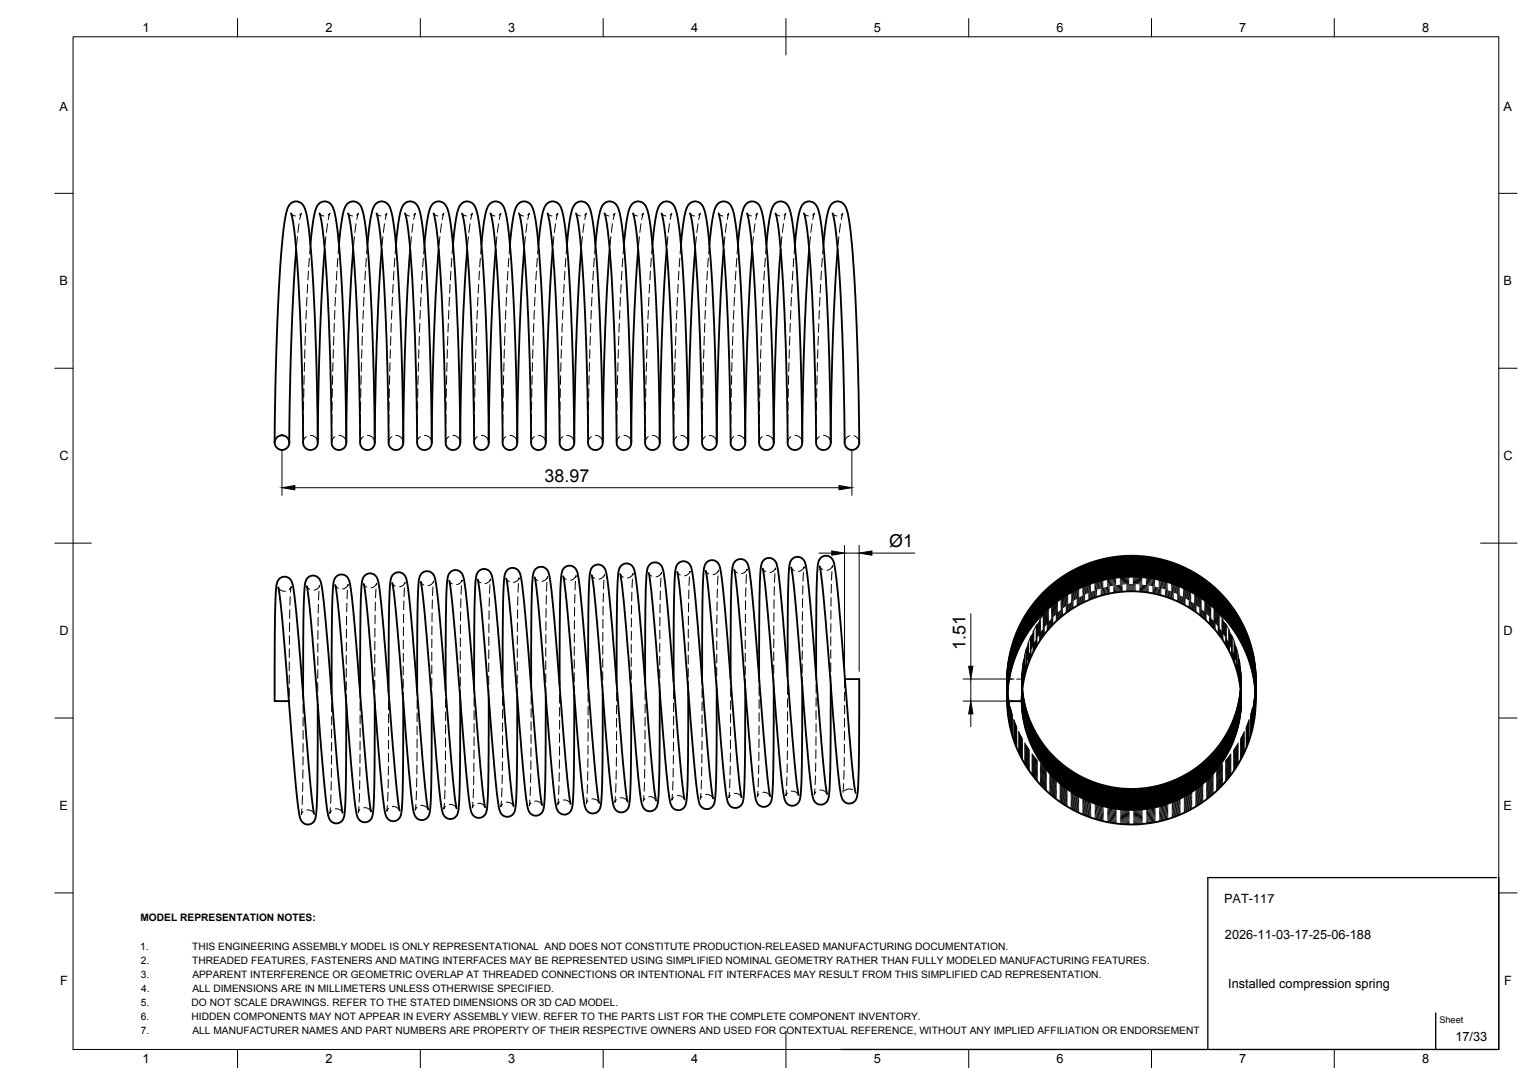
ISO-10303-21;
HEADER;
/* Generated by software containing ST-Developer
 * from STEP Tools, Inc. (www.steptools.com) 
 */

FILE_DESCRIPTION(
/* description */ ('Counterbalanced vertical column'),
/* implementation_level */ '2;1');

FILE_NAME(
/* name */ 'Installed compression spring.step',
/* time_stamp */ '2026-10-29T16:47:22-07:00',
/* author */ (''),
/* organization */ (''),
/* preprocessor_version */ 'ST-DEVELOPER v20.2',
/* originating_system */ 'Autodesk Translation Framework v15.17.0.0',
/* authorisation */ '');

FILE_SCHEMA (('AUTOMOTIVE_DESIGN { 1 0 10303 214 3 1 1 }'));
ENDSEC;

DATA;
#10=MECHANICAL_DESIGN_GEOMETRIC_PRESENTATION_REPRESENTATION('',(#364),#15040);
#278=B_SPLINE_CURVE_WITH_KNOTS('',3,(#13224,#13225,#13226,#13227,#13228,
#13229,#13230,#13231,#13232,#13233,#13234,#13235,#13236,#13237,#13238,#13239,
#13240,#13241,#13242,#13243,#13244,#13245,#13246,#13247,#13248,#13249,#13250,
#13251,#13252,#13253,#13254,#13255,#13256,#13257,#13258,#13259,#13260,#13261,
#13262,#13263,#13264,#13265,#13266,#13267,#13268,#13269,#13270,#13271,#13272,
#13273,#13274,#13275,#13276,#13277,#13278,#13279,#13280,#13281,#13282,#13283,
#13284,#13285,#13286,#13287,#13288,#13289,#13290,#13291,#13292,#13293,#13294,
#13295,#13296,#13297,#13298,#13299,#13300,#13301,#13302,#13303,#13304,#13305,
#13306,#13307,#13308,#13309,#13310,#13311,#13312,#13313,#13314,#13315,#13316,
#13317,#13318,#13319,#13320,#13321,#13322,#13323,#13324,#13325,#13326,#13327,
#13328,#13329,#13330,#13331,#13332,#13333,#13334,#13335,#13336,#13337,#13338,
#13339,#13340,#13341,#13342,#13343,#13344,#13345,#13346,#13347,#13348,#13349,
#13350,#13351,#13352,#13353,#13354,#13355,#13356,#13357,#13358,#13359,#13360,
#13361,#13362,#13363,#13364,#13365,#13366,#13367,#13368,#13369,#13370,#13371,
#13372,#13373,#13374,#13375,#13376,#13377,#13378,#13379,#13380,#13381,#13382,
#13383,#13384,#13385,#13386,#13387,#13388,#13389,#13390,#13391,#13392,#13393,
#13394,#13395,#13396,#13397,#13398,#13399,#13400,#13401,#13402,#13403,#13404,
#13405,#13406,#13407,#13408,#13409,#13410,#13411,#13412,#13413,#13414,#13415,
#13416,#13417,#13418,#13419,#13420,#13421,#13422,#13423,#13424,#13425,#13426,
#13427,#13428,#13429,#13430,#13431,#13432,#13433,#13434,#13435,#13436,#13437,
#13438,#13439,#13440,#13441,#13442,#13443,#13444,#13445,#13446,#13447,#13448,
#13449,#13450,#13451,#13452,#13453,#13454,#13455,#13456,#13457,#13458,#13459,
#13460,#13461,#13462,#13463),.UNSPECIFIED.,.F.,.F.,(4,1,1,1,1,1,1,1,1,1,
1,1,1,1,1,1,1,1,1,1,1,1,1,1,1,1,1,1,1,1,1,1,1,1,1,1,1,1,1,1,1,1,1,1,1,1,
1,1,1,1,1,1,1,1,1,1,1,1,1,1,1,1,1,1,1,1,1,1,1,1,1,1,1,1,1,1,1,1,1,1,1,1,
1,1,1,1,1,1,1,1,1,1,1,1,1,1,1,1,1,1,1,1,1,1,1,1,1,1,1,1,1,1,1,1,1,1,1,1,
1,1,1,1,1,1,1,1,1,1,1,1,1,1,1,1,1,1,1,1,1,1,1,1,1,1,1,1,1,1,1,1,1,1,1,1,
1,1,1,1,1,1,1,1,1,1,1,1,1,1,1,1,1,1,1,1,1,1,1,1,1,1,1,1,1,1,1,1,1,1,1,1,
1,1,1,1,1,1,1,1,1,1,1,1,1,1,1,1,1,1,1,1,1,1,1,1,1,1,1,1,1,1,1,1,1,1,1,1,
1,1,1,1,1,1,1,1,1,1,1,4),(0.,0.00446428571428571,0.00892857142857143,0.0133928571428571,
0.0178571428571429,0.0223214285714286,0.0267857142857143,0.03125,0.0357142857142857,
0.0401785714285714,0.0446428571428571,0.0491071428571428,0.0513392857142857,
0.0535714285714286,0.0580357142857143,0.0625,0.0669642857142857,0.0714285714285714,
0.0758928571428571,0.0803571428571428,0.0848214285714286,0.0892857142857143,
0.09375,0.0982142857142857,0.102678571428571,0.107142857142857,0.111607142857143,
0.116071428571429,0.120535714285714,0.125,0.129464285714286,0.133928571428571,
0.136160714285714,0.138392857142857,0.142857142857143,0.146825396825397,
0.150793650793651,0.154761904761905,0.158730158730159,0.162698412698413,
0.166666666666667,0.170634920634921,0.174603174603175,0.17989417989418,
0.185185185185185,0.19047619047619,0.194444444444444,0.198412698412698,
0.202380952380952,0.206349206349206,0.21031746031746,0.214285714285714,
0.218253968253968,0.220238095238095,0.222222222222222,0.226190476190476,
0.23015873015873,0.234126984126984,0.238095238095238,0.241071428571429,
0.244047619047619,0.247023809523809,0.25,0.25297619047619,0.255952380952381,
0.258928571428571,0.261904761904762,0.267857142857143,0.273809523809524,
0.279761904761905,0.285714285714286,0.291666666666667,0.297619047619048,
0.303571428571429,0.30952380952381,0.31547619047619,0.321428571428571,0.327380952380952,
0.333333333333333,0.339285714285714,0.345238095238095,0.351190476190476,
0.357142857142857,0.363095238095238,0.369047619047619,0.375,0.380952380952381,
0.386904761904762,0.392857142857143,0.398809523809524,0.404761904761905,
0.407738095238095,0.410714285714286,0.413690476190476,0.416666666666667,
0.419642857142857,0.422619047619048,0.425595238095238,0.428571428571429,
0.433035714285714,0.4375,0.441964285714286,0.446428571428571,0.450892857142857,
0.455357142857143,0.459821428571429,0.464285714285714,0.46875,0.473214285714286,
0.477678571428571,0.482142857142857,0.486607142857143,0.491071428571429,
0.495535714285714,0.5,0.504464285714286,0.508928571428571,0.513392857142857,
0.517857142857143,0.522321428571428,0.526785714285714,0.53125,0.535714285714286,
0.540178571428571,0.544642857142857,0.549107142857143,0.553571428571429,
0.558035714285714,0.5625,0.566964285714286,0.571428571428571,0.575892857142857,
0.580357142857143,0.584821428571428,0.589285714285714,0.59375,0.598214285714286,
0.602678571428571,0.607142857142857,0.611607142857143,0.616071428571429,
0.620535714285714,0.625,0.627232142857143,0.629464285714286,0.633928571428571,
0.638392857142857,0.642857142857143,0.645833333333333,0.648809523809524,
0.651785714285714,0.654761904761905,0.657738095238095,0.660714285714286,
0.663690476190476,0.666666666666667,0.66765873015873,0.670634920634921,
0.674603174603175,0.678571428571428,0.683035714285714,0.6875,0.691964285714286,
0.696428571428571,0.700892857142857,0.705357142857143,0.709821428571428,
0.714285714285714,0.717261904761905,0.720238095238095,0.723214285714286,
0.726190476190476,0.729166666666667,0.732142857142857,0.735119047619047,
0.738095238095238,0.744047619047619,0.75,0.755952380952381,0.761904761904762,
0.767857142857143,0.773809523809524,0.779761904761905,0.785714285714286,
0.78968253968254,0.793650793650793,0.797619047619047,0.801587301587302,
0.805555555555555,0.809523809523809,0.8125,0.81547619047619,0.818452380952381,
0.821428571428571,0.824404761904762,0.827380952380952,0.833333333333333,
0.836309523809524,0.839285714285714,0.842261904761905,0.845238095238095,
0.848214285714286,0.851190476190476,0.854166666666667,0.857142857142857,
0.861607142857143,0.866071428571429,0.870535714285714,0.875,0.879464285714286,
0.883928571428571,0.888392857142857,0.892857142857143,0.897321428571428,
0.901785714285714,0.90625,0.910714285714286,0.915178571428571,0.919642857142857,
0.924107142857143,0.928571428571429,0.930803571428571,0.933035714285714,
0.9375,0.941964285714286,0.946428571428571,0.950892857142857,0.955357142857143,
0.959821428571429,0.964285714285714,0.96875,0.973214285714286,0.977678571428572,
0.982142857142857,0.986607142857143,0.991071428571429,0.995535714285714,
1.),.UNSPECIFIED.);
#279=B_SPLINE_SURFACE_WITH_KNOTS('',3,3,((#10821,#10822,#10823,#10824,#10825,
#10826,#10827,#10828,#10829,#10830,#10831,#10832,#10833,#10834,#10835,#10836,
#10837,#10838,#10839,#10840,#10841,#10842,#10843,#10844,#10845,#10846,#10847,
#10848,#10849,#10850,#10851,#10852,#10853,#10854,#10855,#10856,#10857,#10858,
#10859,#10860,#10861,#10862,#10863,#10864,#10865,#10866,#10867,#10868,#10869,
#10870,#10871,#10872,#10873,#10874,#10875,#10876,#10877,#10878,#10879,#10880,
#10881,#10882,#10883,#10884,#10885,#10886,#10887,#10888,#10889,#10890,#10891,
#10892,#10893,#10894,#10895,#10896,#10897,#10898,#10899,#10900,#10901,#10902,
#10903,#10904,#10905,#10906,#10907,#10908,#10909,#10910,#10911,#10912,#10913,
#10914,#10915,#10916,#10917,#10918,#10919,#10920,#10921,#10922,#10923,#10924,
#10925,#10926,#10927,#10928,#10929,#10930,#10931,#10932,#10933,#10934,#10935,
#10936,#10937,#10938,#10939,#10940,#10941,#10942,#10943,#10944,#10945,#10946,
#10947,#10948,#10949,#10950,#10951,#10952,#10953,#10954,#10955,#10956,#10957,
#10958,#10959,#10960,#10961,#10962,#10963,#10964,#10965,#10966,#10967,#10968,
#10969,#10970,#10971,#10972,#10973,#10974,#10975,#10976,#10977,#10978,#10979,
#10980,#10981,#10982,#10983,#10984,#10985,#10986,#10987,#10988,#10989,#10990,
#10991,#10992,#10993,#10994,#10995,#10996,#10997,#10998,#10999,#11000,#11001,
#11002,#11003,#11004,#11005,#11006,#11007,#11008,#11009,#11010,#11011,#11012,
#11013,#11014,#11015,#11016,#11017,#11018,#11019,#11020,#11021,#11022,#11023,
#11024,#11025,#11026,#11027,#11028,#11029,#11030,#11031,#11032,#11033,#11034,
#11035,#11036,#11037,#11038,#11039,#11040,#11041,#11042,#11043,#11044,#11045,
#11046,#11047,#11048,#11049,#11050,#11051,#11052,#11053,#11054,#11055,#11056,
#11057,#11058,#11059,#11060),(#11061,#11062,#11063,#11064,#11065,#11066,
#11067,#11068,#11069,#11070,#11071,#11072,#11073,#11074,#11075,#11076,#11077,
#11078,#11079,#11080,#11081,#11082,#11083,#11084,#11085,#11086,#11087,#11088,
#11089,#11090,#11091,#11092,#11093,#11094,#11095,#11096,#11097,#11098,#11099,
#11100,#11101,#11102,#11103,#11104,#11105,#11106,#11107,#11108,#11109,#11110,
#11111,#11112,#11113,#11114,#11115,#11116,#11117,#11118,#11119,#11120,#11121,
#11122,#11123,#11124,#11125,#11126,#11127,#11128,#11129,#11130,#11131,#11132,
#11133,#11134,#11135,#11136,#11137,#11138,#11139,#11140,#11141,#11142,#11143,
#11144,#11145,#11146,#11147,#11148,#11149,#11150,#11151,#11152,#11153,#11154,
#11155,#11156,#11157,#11158,#11159,#11160,#11161,#11162,#11163,#11164,#11165,
#11166,#11167,#11168,#11169,#11170,#11171,#11172,#11173,#11174,#11175,#11176,
#11177,#11178,#11179,#11180,#11181,#11182,#11183,#11184,#11185,#11186,#11187,
#11188,#11189,#11190,#11191,#11192,#11193,#11194,#11195,#11196,#11197,#11198,
#11199,#11200,#11201,#11202,#11203,#11204,#11205,#11206,#11207,#11208,#11209,
#11210,#11211,#11212,#11213,#11214,#11215,#11216,#11217,#11218,#11219,#11220,
#11221,#11222,#11223,#11224,#11225,#11226,#11227,#11228,#11229,#11230,#11231,
#11232,#11233,#11234,#11235,#11236,#11237,#11238,#11239,#11240,#11241,#11242,
#11243,#11244,#11245,#11246,#11247,#11248,#11249,#11250,#11251,#11252,#11253,
#11254,#11255,#11256,#11257,#11258,#11259,#11260,#11261,#11262,#11263,#11264,
#11265,#11266,#11267,#11268,#11269,#11270,#11271,#11272,#11273,#11274,#11275,
#11276,#11277,#11278,#11279,#11280,#11281,#11282,#11283,#11284,#11285,#11286,
#11287,#11288,#11289,#11290,#11291,#11292,#11293,#11294,#11295,#11296,#11297,
#11298,#11299,#11300),(#11301,#11302,#11303,#11304,#11305,#11306,#11307,
#11308,#11309,#11310,#11311,#11312,#11313,#11314,#11315,#11316,#11317,#11318,
#11319,#11320,#11321,#11322,#11323,#11324,#11325,#11326,#11327,#11328,#11329,
#11330,#11331,#11332,#11333,#11334,#11335,#11336,#11337,#11338,#11339,#11340,
#11341,#11342,#11343,#11344,#11345,#11346,#11347,#11348,#11349,#11350,#11351,
#11352,#11353,#11354,#11355,#11356,#11357,#11358,#11359,#11360,#11361,#11362,
#11363,#11364,#11365,#11366,#11367,#11368,#11369,#11370,#11371,#11372,#11373,
#11374,#11375,#11376,#11377,#11378,#11379,#11380,#11381,#11382,#11383,#11384,
#11385,#11386,#11387,#11388,#11389,#11390,#11391,#11392,#11393,#11394,#11395,
#11396,#11397,#11398,#11399,#11400,#11401,#11402,#11403,#11404,#11405,#11406,
#11407,#11408,#11409,#11410,#11411,#11412,#11413,#11414,#11415,#11416,#11417,
#11418,#11419,#11420,#11421,#11422,#11423,#11424,#11425,#11426,#11427,#11428,
#11429,#11430,#11431,#11432,#11433,#11434,#11435,#11436,#11437,#11438,#11439,
#11440,#11441,#11442,#11443,#11444,#11445,#11446,#11447,#11448,#11449,#11450,
#11451,#11452,#11453,#11454,#11455,#11456,#11457,#11458,#11459,#11460,#11461,
#11462,#11463,#11464,#11465,#11466,#11467,#11468,#11469,#11470,#11471,#11472,
#11473,#11474,#11475,#11476,#11477,#11478,#11479,#11480,#11481,#11482,#11483,
#11484,#11485,#11486,#11487,#11488,#11489,#11490,#11491,#11492,#11493,#11494,
#11495,#11496,#11497,#11498,#11499,#11500,#11501,#11502,#11503,#11504,#11505,
#11506,#11507,#11508,#11509,#11510,#11511,#11512,#11513,#11514,#11515,#11516,
#11517,#11518,#11519,#11520,#11521,#11522,#11523,#11524,#11525,#11526,#11527,
#11528,#11529,#11530,#11531,#11532,#11533,#11534,#11535,#11536,#11537,#11538,
#11539,#11540),(#11541,#11542,#11543,#11544,#11545,#11546,#11547,#11548,
#11549,#11550,#11551,#11552,#11553,#11554,#11555,#11556,#11557,#11558,#11559,
#11560,#11561,#11562,#11563,#11564,#11565,#11566,#11567,#11568,#11569,#11570,
#11571,#11572,#11573,#11574,#11575,#11576,#11577,#11578,#11579,#11580,#11581,
#11582,#11583,#11584,#11585,#11586,#11587,#11588,#11589,#11590,#11591,#11592,
#11593,#11594,#11595,#11596,#11597,#11598,#11599,#11600,#11601,#11602,#11603,
#11604,#11605,#11606,#11607,#11608,#11609,#11610,#11611,#11612,#11613,#11614,
#11615,#11616,#11617,#11618,#11619,#11620,#11621,#11622,#11623,#11624,#11625,
#11626,#11627,#11628,#11629,#11630,#11631,#11632,#11633,#11634,#11635,#11636,
#11637,#11638,#11639,#11640,#11641,#11642,#11643,#11644,#11645,#11646,#11647,
#11648,#11649,#11650,#11651,#11652,#11653,#11654,#11655,#11656,#11657,#11658,
#11659,#11660,#11661,#11662,#11663,#11664,#11665,#11666,#11667,#11668,#11669,
#11670,#11671,#11672,#11673,#11674,#11675,#11676,#11677,#11678,#11679,#11680,
#11681,#11682,#11683,#11684,#11685,#11686,#11687,#11688,#11689,#11690,#11691,
#11692,#11693,#11694,#11695,#11696,#11697,#11698,#11699,#11700,#11701,#11702,
#11703,#11704,#11705,#11706,#11707,#11708,#11709,#11710,#11711,#11712,#11713,
#11714,#11715,#11716,#11717,#11718,#11719,#11720,#11721,#11722,#11723,#11724,
#11725,#11726,#11727,#11728,#11729,#11730,#11731,#11732,#11733,#11734,#11735,
#11736,#11737,#11738,#11739,#11740,#11741,#11742,#11743,#11744,#11745,#11746,
#11747,#11748,#11749,#11750,#11751,#11752,#11753,#11754,#11755,#11756,#11757,
#11758,#11759,#11760,#11761,#11762,#11763,#11764,#11765,#11766,#11767,#11768,
#11769,#11770,#11771,#11772,#11773,#11774,#11775,#11776,#11777,#11778,#11779,
#11780),(#11781,#11782,#11783,#11784,#11785,#11786,#11787,#11788,#11789,
#11790,#11791,#11792,#11793,#11794,#11795,#11796,#11797,#11798,#11799,#11800,
#11801,#11802,#11803,#11804,#11805,#11806,#11807,#11808,#11809,#11810,#11811,
#11812,#11813,#11814,#11815,#11816,#11817,#11818,#11819,#11820,#11821,#11822,
#11823,#11824,#11825,#11826,#11827,#11828,#11829,#11830,#11831,#11832,#11833,
#11834,#11835,#11836,#11837,#11838,#11839,#11840,#11841,#11842,#11843,#11844,
#11845,#11846,#11847,#11848,#11849,#11850,#11851,#11852,#11853,#11854,#11855,
#11856,#11857,#11858,#11859,#11860,#11861,#11862,#11863,#11864,#11865,#11866,
#11867,#11868,#11869,#11870,#11871,#11872,#11873,#11874,#11875,#11876,#11877,
#11878,#11879,#11880,#11881,#11882,#11883,#11884,#11885,#11886,#11887,#11888,
#11889,#11890,#11891,#11892,#11893,#11894,#11895,#11896,#11897,#11898,#11899,
#11900,#11901,#11902,#11903,#11904,#11905,#11906,#11907,#11908,#11909,#11910,
#11911,#11912,#11913,#11914,#11915,#11916,#11917,#11918,#11919,#11920,#11921,
#11922,#11923,#11924,#11925,#11926,#11927,#11928,#11929,#11930,#11931,#11932,
#11933,#11934,#11935,#11936,#11937,#11938,#11939,#11940,#11941,#11942,#11943,
#11944,#11945,#11946,#11947,#11948,#11949,#11950,#11951,#11952,#11953,#11954,
#11955,#11956,#11957,#11958,#11959,#11960,#11961,#11962,#11963,#11964,#11965,
#11966,#11967,#11968,#11969,#11970,#11971,#11972,#11973,#11974,#11975,#11976,
#11977,#11978,#11979,#11980,#11981,#11982,#11983,#11984,#11985,#11986,#11987,
#11988,#11989,#11990,#11991,#11992,#11993,#11994,#11995,#11996,#11997,#11998,
#11999,#12000,#12001,#12002,#12003,#12004,#12005,#12006,#12007,#12008,#12009,
#12010,#12011,#12012,#12013,#12014,#12015,#12016,#12017,#12018,#12019,#12020),
(#12021,#12022,#12023,#12024,#12025,#12026,#12027,#12028,#12029,#12030,
#12031,#12032,#12033,#12034,#12035,#12036,#12037,#12038,#12039,#12040,#12041,
#12042,#12043,#12044,#12045,#12046,#12047,#12048,#12049,#12050,#12051,#12052,
#12053,#12054,#12055,#12056,#12057,#12058,#12059,#12060,#12061,#12062,#12063,
#12064,#12065,#12066,#12067,#12068,#12069,#12070,#12071,#12072,#12073,#12074,
#12075,#12076,#12077,#12078,#12079,#12080,#12081,#12082,#12083,#12084,#12085,
#12086,#12087,#12088,#12089,#12090,#12091,#12092,#12093,#12094,#12095,#12096,
#12097,#12098,#12099,#12100,#12101,#12102,#12103,#12104,#12105,#12106,#12107,
#12108,#12109,#12110,#12111,#12112,#12113,#12114,#12115,#12116,#12117,#12118,
#12119,#12120,#12121,#12122,#12123,#12124,#12125,#12126,#12127,#12128,#12129,
#12130,#12131,#12132,#12133,#12134,#12135,#12136,#12137,#12138,#12139,#12140,
#12141,#12142,#12143,#12144,#12145,#12146,#12147,#12148,#12149,#12150,#12151,
#12152,#12153,#12154,#12155,#12156,#12157,#12158,#12159,#12160,#12161,#12162,
#12163,#12164,#12165,#12166,#12167,#12168,#12169,#12170,#12171,#12172,#12173,
#12174,#12175,#12176,#12177,#12178,#12179,#12180,#12181,#12182,#12183,#12184,
#12185,#12186,#12187,#12188,#12189,#12190,#12191,#12192,#12193,#12194,#12195,
#12196,#12197,#12198,#12199,#12200,#12201,#12202,#12203,#12204,#12205,#12206,
#12207,#12208,#12209,#12210,#12211,#12212,#12213,#12214,#12215,#12216,#12217,
#12218,#12219,#12220,#12221,#12222,#12223,#12224,#12225,#12226,#12227,#12228,
#12229,#12230,#12231,#12232,#12233,#12234,#12235,#12236,#12237,#12238,#12239,
#12240,#12241,#12242,#12243,#12244,#12245,#12246,#12247,#12248,#12249,#12250,
#12251,#12252,#12253,#12254,#12255,#12256,#12257,#12258,#12259,#12260),
(#12261,#12262,#12263,#12264,#12265,#12266,#12267,#12268,#12269,#12270,
#12271,#12272,#12273,#12274,#12275,#12276,#12277,#12278,#12279,#12280,#12281,
#12282,#12283,#12284,#12285,#12286,#12287,#12288,#12289,#12290,#12291,#12292,
#12293,#12294,#12295,#12296,#12297,#12298,#12299,#12300,#12301,#12302,#12303,
#12304,#12305,#12306,#12307,#12308,#12309,#12310,#12311,#12312,#12313,#12314,
#12315,#12316,#12317,#12318,#12319,#12320,#12321,#12322,#12323,#12324,#12325,
#12326,#12327,#12328,#12329,#12330,#12331,#12332,#12333,#12334,#12335,#12336,
#12337,#12338,#12339,#12340,#12341,#12342,#12343,#12344,#12345,#12346,#12347,
#12348,#12349,#12350,#12351,#12352,#12353,#12354,#12355,#12356,#12357,#12358,
#12359,#12360,#12361,#12362,#12363,#12364,#12365,#12366,#12367,#12368,#12369,
#12370,#12371,#12372,#12373,#12374,#12375,#12376,#12377,#12378,#12379,#12380,
#12381,#12382,#12383,#12384,#12385,#12386,#12387,#12388,#12389,#12390,#12391,
#12392,#12393,#12394,#12395,#12396,#12397,#12398,#12399,#12400,#12401,#12402,
#12403,#12404,#12405,#12406,#12407,#12408,#12409,#12410,#12411,#12412,#12413,
#12414,#12415,#12416,#12417,#12418,#12419,#12420,#12421,#12422,#12423,#12424,
#12425,#12426,#12427,#12428,#12429,#12430,#12431,#12432,#12433,#12434,#12435,
#12436,#12437,#12438,#12439,#12440,#12441,#12442,#12443,#12444,#12445,#12446,
#12447,#12448,#12449,#12450,#12451,#12452,#12453,#12454,#12455,#12456,#12457,
#12458,#12459,#12460,#12461,#12462,#12463,#12464,#12465,#12466,#12467,#12468,
#12469,#12470,#12471,#12472,#12473,#12474,#12475,#12476,#12477,#12478,#12479,
#12480,#12481,#12482,#12483,#12484,#12485,#12486,#12487,#12488,#12489,#12490,
#12491,#12492,#12493,#12494,#12495,#12496,#12497,#12498,#12499,#12500),
(#12501,#12502,#12503,#12504,#12505,#12506,#12507,#12508,#12509,#12510,
#12511,#12512,#12513,#12514,#12515,#12516,#12517,#12518,#12519,#12520,#12521,
#12522,#12523,#12524,#12525,#12526,#12527,#12528,#12529,#12530,#12531,#12532,
#12533,#12534,#12535,#12536,#12537,#12538,#12539,#12540,#12541,#12542,#12543,
#12544,#12545,#12546,#12547,#12548,#12549,#12550,#12551,#12552,#12553,#12554,
#12555,#12556,#12557,#12558,#12559,#12560,#12561,#12562,#12563,#12564,#12565,
#12566,#12567,#12568,#12569,#12570,#12571,#12572,#12573,#12574,#12575,#12576,
#12577,#12578,#12579,#12580,#12581,#12582,#12583,#12584,#12585,#12586,#12587,
#12588,#12589,#12590,#12591,#12592,#12593,#12594,#12595,#12596,#12597,#12598,
#12599,#12600,#12601,#12602,#12603,#12604,#12605,#12606,#12607,#12608,#12609,
#12610,#12611,#12612,#12613,#12614,#12615,#12616,#12617,#12618,#12619,#12620,
#12621,#12622,#12623,#12624,#12625,#12626,#12627,#12628,#12629,#12630,#12631,
#12632,#12633,#12634,#12635,#12636,#12637,#12638,#12639,#12640,#12641,#12642,
#12643,#12644,#12645,#12646,#12647,#12648,#12649,#12650,#12651,#12652,#12653,
#12654,#12655,#12656,#12657,#12658,#12659,#12660,#12661,#12662,#12663,#12664,
#12665,#12666,#12667,#12668,#12669,#12670,#12671,#12672,#12673,#12674,#12675,
#12676,#12677,#12678,#12679,#12680,#12681,#12682,#12683,#12684,#12685,#12686,
#12687,#12688,#12689,#12690,#12691,#12692,#12693,#12694,#12695,#12696,#12697,
#12698,#12699,#12700,#12701,#12702,#12703,#12704,#12705,#12706,#12707,#12708,
#12709,#12710,#12711,#12712,#12713,#12714,#12715,#12716,#12717,#12718,#12719,
#12720,#12721,#12722,#12723,#12724,#12725,#12726,#12727,#12728,#12729,#12730,
#12731,#12732,#12733,#12734,#12735,#12736,#12737,#12738,#12739,#12740),
(#12741,#12742,#12743,#12744,#12745,#12746,#12747,#12748,#12749,#12750,
#12751,#12752,#12753,#12754,#12755,#12756,#12757,#12758,#12759,#12760,#12761,
#12762,#12763,#12764,#12765,#12766,#12767,#12768,#12769,#12770,#12771,#12772,
#12773,#12774,#12775,#12776,#12777,#12778,#12779,#12780,#12781,#12782,#12783,
#12784,#12785,#12786,#12787,#12788,#12789,#12790,#12791,#12792,#12793,#12794,
#12795,#12796,#12797,#12798,#12799,#12800,#12801,#12802,#12803,#12804,#12805,
#12806,#12807,#12808,#12809,#12810,#12811,#12812,#12813,#12814,#12815,#12816,
#12817,#12818,#12819,#12820,#12821,#12822,#12823,#12824,#12825,#12826,#12827,
#12828,#12829,#12830,#12831,#12832,#12833,#12834,#12835,#12836,#12837,#12838,
#12839,#12840,#12841,#12842,#12843,#12844,#12845,#12846,#12847,#12848,#12849,
#12850,#12851,#12852,#12853,#12854,#12855,#12856,#12857,#12858,#12859,#12860,
#12861,#12862,#12863,#12864,#12865,#12866,#12867,#12868,#12869,#12870,#12871,
#12872,#12873,#12874,#12875,#12876,#12877,#12878,#12879,#12880,#12881,#12882,
#12883,#12884,#12885,#12886,#12887,#12888,#12889,#12890,#12891,#12892,#12893,
#12894,#12895,#12896,#12897,#12898,#12899,#12900,#12901,#12902,#12903,#12904,
#12905,#12906,#12907,#12908,#12909,#12910,#12911,#12912,#12913,#12914,#12915,
#12916,#12917,#12918,#12919,#12920,#12921,#12922,#12923,#12924,#12925,#12926,
#12927,#12928,#12929,#12930,#12931,#12932,#12933,#12934,#12935,#12936,#12937,
#12938,#12939,#12940,#12941,#12942,#12943,#12944,#12945,#12946,#12947,#12948,
#12949,#12950,#12951,#12952,#12953,#12954,#12955,#12956,#12957,#12958,#12959,
#12960,#12961,#12962,#12963,#12964,#12965,#12966,#12967,#12968,#12969,#12970,
#12971,#12972,#12973,#12974,#12975,#12976,#12977,#12978,#12979,#12980),
(#12981,#12982,#12983,#12984,#12985,#12986,#12987,#12988,#12989,#12990,
#12991,#12992,#12993,#12994,#12995,#12996,#12997,#12998,#12999,#13000,#13001,
#13002,#13003,#13004,#13005,#13006,#13007,#13008,#13009,#13010,#13011,#13012,
#13013,#13014,#13015,#13016,#13017,#13018,#13019,#13020,#13021,#13022,#13023,
#13024,#13025,#13026,#13027,#13028,#13029,#13030,#13031,#13032,#13033,#13034,
#13035,#13036,#13037,#13038,#13039,#13040,#13041,#13042,#13043,#13044,#13045,
#13046,#13047,#13048,#13049,#13050,#13051,#13052,#13053,#13054,#13055,#13056,
#13057,#13058,#13059,#13060,#13061,#13062,#13063,#13064,#13065,#13066,#13067,
#13068,#13069,#13070,#13071,#13072,#13073,#13074,#13075,#13076,#13077,#13078,
#13079,#13080,#13081,#13082,#13083,#13084,#13085,#13086,#13087,#13088,#13089,
#13090,#13091,#13092,#13093,#13094,#13095,#13096,#13097,#13098,#13099,#13100,
#13101,#13102,#13103,#13104,#13105,#13106,#13107,#13108,#13109,#13110,#13111,
#13112,#13113,#13114,#13115,#13116,#13117,#13118,#13119,#13120,#13121,#13122,
#13123,#13124,#13125,#13126,#13127,#13128,#13129,#13130,#13131,#13132,#13133,
#13134,#13135,#13136,#13137,#13138,#13139,#13140,#13141,#13142,#13143,#13144,
#13145,#13146,#13147,#13148,#13149,#13150,#13151,#13152,#13153,#13154,#13155,
#13156,#13157,#13158,#13159,#13160,#13161,#13162,#13163,#13164,#13165,#13166,
#13167,#13168,#13169,#13170,#13171,#13172,#13173,#13174,#13175,#13176,#13177,
#13178,#13179,#13180,#13181,#13182,#13183,#13184,#13185,#13186,#13187,#13188,
#13189,#13190,#13191,#13192,#13193,#13194,#13195,#13196,#13197,#13198,#13199,
#13200,#13201,#13202,#13203,#13204,#13205,#13206,#13207,#13208,#13209,#13210,
#13211,#13212,#13213,#13214,#13215,#13216,#13217,#13218,#13219,#13220)),
 .UNSPECIFIED.,.T.,.F.,.F.,(4,1,1,1,1,1,1,4),(4,1,1,1,1,1,1,1,1,1,1,1,1,
1,1,1,1,1,1,1,1,1,1,1,1,1,1,1,1,1,1,1,1,1,1,1,1,1,1,1,1,1,1,1,1,1,1,1,1,
1,1,1,1,1,1,1,1,1,1,1,1,1,1,1,1,1,1,1,1,1,1,1,1,1,1,1,1,1,1,1,1,1,1,1,1,
1,1,1,1,1,1,1,1,1,1,1,1,1,1,1,1,1,1,1,1,1,1,1,1,1,1,1,1,1,1,1,1,1,1,1,1,
1,1,1,1,1,1,1,1,1,1,1,1,1,1,1,1,1,1,1,1,1,1,1,1,1,1,1,1,1,1,1,1,1,1,1,1,
1,1,1,1,1,1,1,1,1,1,1,1,1,1,1,1,1,1,1,1,1,1,1,1,1,1,1,1,1,1,1,1,1,1,1,1,
1,1,1,1,1,1,1,1,1,1,1,1,1,1,1,1,1,1,1,1,1,1,1,1,1,1,1,1,1,1,1,1,1,1,1,1,
1,1,1,1,1,1,1,1,4),(-3.14159265358979,-2.24399475256414,-1.34639685153848,
-0.448798950512828,0.448798950512828,1.34639685153848,2.24399475256414,
3.14159265358979),(0.,0.00446428571428571,0.00892857142857143,0.0133928571428571,
0.0178571428571429,0.0223214285714286,0.0267857142857143,0.03125,0.0357142857142857,
0.0401785714285714,0.0446428571428571,0.0491071428571428,0.0513392857142857,
0.0535714285714286,0.0580357142857143,0.0625,0.0669642857142857,0.0714285714285714,
0.0758928571428571,0.0803571428571428,0.0848214285714286,0.0892857142857143,
0.09375,0.0982142857142857,0.102678571428571,0.107142857142857,0.111607142857143,
0.116071428571429,0.120535714285714,0.125,0.129464285714286,0.133928571428571,
0.136160714285714,0.138392857142857,0.142857142857143,0.146825396825397,
0.150793650793651,0.154761904761905,0.158730158730159,0.162698412698413,
0.166666666666667,0.170634920634921,0.174603174603175,0.17989417989418,
0.185185185185185,0.19047619047619,0.194444444444444,0.198412698412698,
0.202380952380952,0.206349206349206,0.21031746031746,0.214285714285714,
0.218253968253968,0.220238095238095,0.222222222222222,0.226190476190476,
0.23015873015873,0.234126984126984,0.238095238095238,0.241071428571429,
0.244047619047619,0.247023809523809,0.25,0.25297619047619,0.255952380952381,
0.258928571428571,0.261904761904762,0.267857142857143,0.273809523809524,
0.279761904761905,0.285714285714286,0.291666666666667,0.297619047619048,
0.303571428571429,0.30952380952381,0.31547619047619,0.321428571428571,0.327380952380952,
0.333333333333333,0.339285714285714,0.345238095238095,0.351190476190476,
0.357142857142857,0.363095238095238,0.369047619047619,0.375,0.380952380952381,
0.386904761904762,0.392857142857143,0.398809523809524,0.404761904761905,
0.407738095238095,0.410714285714286,0.413690476190476,0.416666666666667,
0.419642857142857,0.422619047619048,0.425595238095238,0.428571428571429,
0.433035714285714,0.4375,0.441964285714286,0.446428571428571,0.450892857142857,
0.455357142857143,0.459821428571429,0.464285714285714,0.46875,0.473214285714286,
0.477678571428571,0.482142857142857,0.486607142857143,0.491071428571429,
0.495535714285714,0.5,0.504464285714286,0.508928571428571,0.513392857142857,
0.517857142857143,0.522321428571428,0.526785714285714,0.53125,0.535714285714286,
0.540178571428571,0.544642857142857,0.549107142857143,0.553571428571429,
0.558035714285714,0.5625,0.566964285714286,0.571428571428571,0.575892857142857,
0.580357142857143,0.584821428571428,0.589285714285714,0.59375,0.598214285714286,
0.602678571428571,0.607142857142857,0.611607142857143,0.616071428571429,
0.620535714285714,0.625,0.627232142857143,0.629464285714286,0.633928571428571,
0.638392857142857,0.642857142857143,0.645833333333333,0.648809523809524,
0.651785714285714,0.654761904761905,0.657738095238095,0.660714285714286,
0.663690476190476,0.666666666666667,0.66765873015873,0.670634920634921,
0.674603174603175,0.678571428571428,0.683035714285714,0.6875,0.691964285714286,
0.696428571428571,0.700892857142857,0.705357142857143,0.709821428571428,
0.714285714285714,0.717261904761905,0.720238095238095,0.723214285714286,
0.726190476190476,0.729166666666667,0.732142857142857,0.735119047619047,
0.738095238095238,0.744047619047619,0.75,0.755952380952381,0.761904761904762,
0.767857142857143,0.773809523809524,0.779761904761905,0.785714285714286,
0.78968253968254,0.793650793650793,0.797619047619047,0.801587301587302,
0.805555555555555,0.809523809523809,0.8125,0.81547619047619,0.818452380952381,
0.821428571428571,0.824404761904762,0.827380952380952,0.833333333333333,
0.836309523809524,0.839285714285714,0.842261904761905,0.845238095238095,
0.848214285714286,0.851190476190476,0.854166666666667,0.857142857142857,
0.861607142857143,0.866071428571429,0.870535714285714,0.875,0.879464285714286,
0.883928571428571,0.888392857142857,0.892857142857143,0.897321428571428,
0.901785714285714,0.90625,0.910714285714286,0.915178571428571,0.919642857142857,
0.924107142857143,0.928571428571429,0.930803571428571,0.933035714285714,
0.9375,0.941964285714286,0.946428571428571,0.950892857142857,0.955357142857143,
0.959821428571429,0.964285714285714,0.96875,0.973214285714286,0.977678571428572,
0.982142857142857,0.986607142857143,0.991071428571429,0.995535714285714,
1.),.UNSPECIFIED.);
#294=SHAPE_REPRESENTATION_RELATIONSHIP('SRR','None',#15198,#329);
#329=ADVANCED_BREP_SHAPE_REPRESENTATION('',(#399),#15017);
#364=STYLED_ITEM('',(#15457),#399);
#399=MANIFOLD_SOLID_BREP('Body1',#7087);
#603=PLANE('',#7706);
#604=PLANE('',#7707);
#937=FACE_OUTER_BOUND('',#1394,.T.);
#938=FACE_OUTER_BOUND('',#1395,.T.);
#939=FACE_OUTER_BOUND('',#1396,.T.);
#1394=EDGE_LOOP('',(#5214,#5215,#5216,#5217));
#1395=EDGE_LOOP('',(#5218));
#1396=EDGE_LOOP('',(#5219));
#3171=CIRCLE('',#7704,0.05);
#3172=CIRCLE('',#7705,0.05);
#3448=VERTEX_POINT('',#13221);
#3449=VERTEX_POINT('',#13223);
#4108=EDGE_CURVE('',#3448,#3448,#3171,.T.);
#4109=EDGE_CURVE('',#3448,#3449,#278,.T.);
#4110=EDGE_CURVE('',#3449,#3449,#3172,.T.);
#5214=ORIENTED_EDGE('',*,*,#4108,.T.);
#5215=ORIENTED_EDGE('',*,*,#4109,.T.);
#5216=ORIENTED_EDGE('',*,*,#4110,.F.);
#5217=ORIENTED_EDGE('',*,*,#4109,.F.);
#5218=ORIENTED_EDGE('',*,*,#4110,.T.);
#5219=ORIENTED_EDGE('',*,*,#4108,.F.);
#6779=ADVANCED_FACE('',(#937),#279,.T.);
#6780=ADVANCED_FACE('',(#938),#603,.T.);
#6781=ADVANCED_FACE('',(#939),#604,.F.);
#7087=CLOSED_SHELL('',(#6779,#6780,#6781));
#7703=AXIS2_PLACEMENT_3D('',#10820,#8766,#8767);
#7704=AXIS2_PLACEMENT_3D('',#13222,#8768,#8769);
#7705=AXIS2_PLACEMENT_3D('',#13464,#8770,#8771);
#7706=AXIS2_PLACEMENT_3D('',#13465,#8772,#8773);
#7707=AXIS2_PLACEMENT_3D('',#13466,#8774,#8775);
#8766=DIRECTION('axis',(0.,0.,1.));
#8767=DIRECTION('refdir',(1.,0.,0.));
#8768=DIRECTION('center_axis',(-0.00013439580876317,0.999252824179506,0.0386493894783381));
#8769=DIRECTION('ref_axis',(5.19819987946072E-6,-0.0386493891287688,0.999252833217375));
#8770=DIRECTION('center_axis',(0.000134396360781948,0.999252824161965,0.0386493899299144));
#8771=DIRECTION('ref_axis',(0.987395345410578,-0.00624976689623724,0.158149841211642));
#8772=DIRECTION('center_axis',(0.000134396360781948,0.999252824161965,0.0386493899299144));
#8773=DIRECTION('ref_axis',(0.987395345410578,-0.00624976689623724,0.158149841211642));
#8774=DIRECTION('center_axis',(-0.00013439580876317,0.999252824179506,0.0386493894783381));
#8775=DIRECTION('ref_axis',(5.19819987946073E-6,-0.0386493891287688,0.999252833217375));
#10820=CARTESIAN_POINT('',(0.,0.,0.));
#10821=CARTESIAN_POINT('Ctrl Pts',(-6.20000025990999,0.00193246945643844,
1.00003735833913));
#10822=CARTESIAN_POINT('Ctrl Pts',(-6.20002044487095,0.15201065585541,1.00584212579936));
#10823=CARTESIAN_POINT('Ctrl Pts',(-6.28611355781982,0.450654413607575,
1.01745595262984));
#10824=CARTESIAN_POINT('Ctrl Pts',(-6.63487773043299,0.762776896374944,
1.0349026678303));
#10825=CARTESIAN_POINT('Ctrl Pts',(-7.09661480461016,0.841046944166038,
1.05237210147879));
#10826=CARTESIAN_POINT('Ctrl Pts',(-7.5301000809641,0.66191148032223,1.06986555847399));
#10827=CARTESIAN_POINT('Ctrl Pts',(-7.8019176387512,0.278705057923738,1.08738232429735));
#10828=CARTESIAN_POINT('Ctrl Pts',(-7.82838413701279,-0.19084760704926,
1.10492270302733));
#10829=CARTESIAN_POINT('Ctrl Pts',(-7.60064075566285,-0.603137091155931,
1.12248646715818));
#10830=CARTESIAN_POINT('Ctrl Pts',(-7.1879122444388,-0.831327694844811,
1.1400736154085));
#10831=CARTESIAN_POINT('Ctrl Pts',(-6.71648331627183,-0.804952825733149,
1.15768402928987));
#10832=CARTESIAN_POINT('Ctrl Pts',(-6.33069129380762,-0.53139586788873,
1.17531762920689));
#10833=CARTESIAN_POINT('Ctrl Pts',(-6.17986938434826,-0.166924530929506,
1.19003152205635));
#10834=CARTESIAN_POINT('Ctrl Pts',(-6.18891827393114,0.139694417819641,
1.20181411747366));
#10835=CARTESIAN_POINT('Ctrl Pts',(-6.28167759636603,0.432287479563812,
1.21360434390419));
#10836=CARTESIAN_POINT('Ctrl Pts',(-6.54498491257115,0.727352514001043,
1.22835639528026));
#10837=CARTESIAN_POINT('Ctrl Pts',(-7.00178799837524,0.858989074734809,
1.2460815491715));
#10838=CARTESIAN_POINT('Ctrl Pts',(-7.45905640505002,0.727341633611197,
1.2638292469814));
#10839=CARTESIAN_POINT('Ctrl Pts',(-7.77665281049733,0.372097321399229,
1.28159932797245));
#10840=CARTESIAN_POINT('Ctrl Pts',(-7.85663990835041,-0.0982374580424732,
1.29939162334549));
#10841=CARTESIAN_POINT('Ctrl Pts',(-7.67391806687674,-0.539592338752092,
1.31720595246947));
#10842=CARTESIAN_POINT('Ctrl Pts',(-7.28390423314539,-0.816419475206943,
1.33504212338853));
#10843=CARTESIAN_POINT('Ctrl Pts',(-6.80581165670056,-0.843349744908527,
1.35289993632842));
#10844=CARTESIAN_POINT('Ctrl Pts',(-6.38616737126169,-0.61151281975725,
1.37077917836497));
#10845=CARTESIAN_POINT('Ctrl Pts',(-6.15391471330266,-0.191448545046746,
1.38867962991899));
#10846=CARTESIAN_POINT('Ctrl Pts',(-6.18078031189829,0.288356063072798,
1.40660105660474));
#10847=CARTESIAN_POINT('Ctrl Pts',(-6.45912099114284,0.680780452257456,
1.42454321935777));
#10848=CARTESIAN_POINT('Ctrl Pts',(-6.90408886634936,0.865172061566579,
1.44250586618275));
#10849=CARTESIAN_POINT('Ctrl Pts',(-7.37948719351768,0.784486199243698,
1.46048873474343));
#10850=CARTESIAN_POINT('Ctrl Pts',(-7.73949168252554,0.462850086060547,
1.47849155669373));
#10851=CARTESIAN_POINT('Ctrl Pts',(-7.87332738631526,-0.0014557841833066,
1.49651404939771));
#10852=CARTESIAN_POINT('Ctrl Pts',(-7.73949699110486,-0.466462821459191,
1.51455592727214));
#10853=CARTESIAN_POINT('Ctrl Pts',(-7.43853082628792,-0.735208997602771,
1.52960672657187));
#10854=CARTESIAN_POINT('Ctrl Pts',(-7.13950426621928,-0.830029799823059,
1.5416567556677));
#10855=CARTESIAN_POINT('Ctrl Pts',(-6.82573429908325,-0.839341203501555,
1.55371299076107));
#10856=CARTESIAN_POINT('Ctrl Pts',(-6.46884268588545,-0.691631510671627,
1.56812451918729));
#10857=CARTESIAN_POINT('Ctrl Pts',(-6.19953260950331,-0.335836989319061,
1.58489796930832));
#10858=CARTESIAN_POINT('Ctrl Pts',(-6.13558329245919,0.087838843174565,
1.60101457637617));
#10859=CARTESIAN_POINT('Ctrl Pts',(-6.28224419701691,0.490989051876738,
1.61714503893002));
#10860=CARTESIAN_POINT('Ctrl Pts',(-6.60413478737033,0.775061465279082,
1.63328911262099));
#10861=CARTESIAN_POINT('Ctrl Pts',(-7.02294084448011,0.870730250827747,
1.64944654818199));
#10862=CARTESIAN_POINT('Ctrl Pts',(-7.43707348216018,0.754258049077075,
1.66561709103637));
#10863=CARTESIAN_POINT('Ctrl Pts',(-7.74477169774561,0.453838654047166,
1.68180048156974));
#10864=CARTESIAN_POINT('Ctrl Pts',(-7.88680288613318,-0.003482702933719,
1.69979600813884));
#10865=CARTESIAN_POINT('Ctrl Pts',(-7.73694295256561,-0.521688074393446,
1.71960864643413));
#10866=CARTESIAN_POINT('Ctrl Pts',(-7.2579246797109,-0.866176668338957,
1.74124367709995));
#10867=CARTESIAN_POINT('Ctrl Pts',(-6.71798257071652,-0.843361624137061,
1.76109465157299));
#10868=CARTESIAN_POINT('Ctrl Pts',(-6.32813840204838,-0.562067108424238,
1.779155502939));
#10869=CARTESIAN_POINT('Ctrl Pts',(-6.1403602470473,-0.172779460138823,
1.79542117132473));
#10870=CARTESIAN_POINT('Ctrl Pts',(-6.16191594592092,0.259681676239064,
1.81169744765855));
#10871=CARTESIAN_POINT('Ctrl Pts',(-6.38773509477738,0.629211178523826,
1.82798403284572));
#10872=CARTESIAN_POINT('Ctrl Pts',(-6.76298297690006,0.845905336791279,
1.84428062449289));
#10873=CARTESIAN_POINT('Ctrl Pts',(-7.1966047520639,0.856877177797125,1.86058691436274));
#10874=CARTESIAN_POINT('Ctrl Pts',(-7.51813159987616,0.691704323104765,
1.87418331464002));
#10875=CARTESIAN_POINT('Ctrl Pts',(-7.70496340534196,0.479537214773933,
1.88506497141452));
#10876=CARTESIAN_POINT('Ctrl Pts',(-7.834243376472,0.228058843588403,1.89594960161061));
#10877=CARTESIAN_POINT('Ctrl Pts',(-7.87040214071621,-0.132058080538115,
1.90956086256863));
#10878=CARTESIAN_POINT('Ctrl Pts',(-7.70176729712619,-0.532544739489079,
1.92590281458038));
#10879=CARTESIAN_POINT('Ctrl Pts',(-7.3617541753632,-0.803795766305812,
1.94225288140178));
#10880=CARTESIAN_POINT('Ctrl Pts',(-6.96910081682361,-0.872691342258758,
1.95724758038991));
#10881=CARTESIAN_POINT('Ctrl Pts',(-6.62358365553027,-0.779878922686934,
1.97088456464667));
#10882=CARTESIAN_POINT('Ctrl Pts',(-6.36438571820951,-0.588772954661729,
1.98316190508021));
#10883=CARTESIAN_POINT('Ctrl Pts',(-6.19306544459119,-0.315928048614165,
1.99544316011942));
#10884=CARTESIAN_POINT('Ctrl Pts',(-6.13303928680132,0.000731296674565001,
2.00772818860116));
#10885=CARTESIAN_POINT('Ctrl Pts',(-6.19306246181983,0.31737131710264,2.02001684693935));
#10886=CARTESIAN_POINT('Ctrl Pts',(-6.36452596264878,0.590662777058206,
2.03230899246722));
#10887=CARTESIAN_POINT('Ctrl Pts',(-6.62407285476001,0.781608449704824,
2.04460448181281));
#10888=CARTESIAN_POINT('Ctrl Pts',(-7.03960726862712,0.894452101215339,
2.06100273047082));
#10889=CARTESIAN_POINT('Ctrl Pts',(-7.58098213708746,0.728278840923384,
2.08150817561209));
#10890=CARTESIAN_POINT('Ctrl Pts',(-7.9216670182819,0.138324035331395,2.10612575173056));
#10891=CARTESIAN_POINT('Ctrl Pts',(-7.77006105183817,-0.525438678362505,
2.13075319116009));
#10892=CARTESIAN_POINT('Ctrl Pts',(-7.20723620509449,-0.909325593088126,
2.15538930422495));
#10893=CARTESIAN_POINT('Ctrl Pts',(-6.53333888373858,-0.807749099412924,
2.18003289797092));
#10894=CARTESIAN_POINT('Ctrl Pts',(-6.1083188432114,-0.274839326778277,
2.204682767912));
#10895=CARTESIAN_POINT('Ctrl Pts',(-6.15924265883207,0.405062095085805,
2.22933770998693));
#10896=CARTESIAN_POINT('Ctrl Pts',(-6.65910391363797,0.868885188693027,
2.25399651054932));
#10897=CARTESIAN_POINT('Ctrl Pts',(-7.34108037988483,0.868897827671466,
2.2786579570982));
#10898=CARTESIAN_POINT('Ctrl Pts',(-7.84103724749041,0.405011680967366,
2.30332083156262));
#10899=CARTESIAN_POINT('Ctrl Pts',(-7.89200269882987,-0.275103355231245,
2.32798391722886));
#10900=CARTESIAN_POINT('Ctrl Pts',(-7.46677961363602,-0.808302976870588,
2.35264599503351));
#10901=CARTESIAN_POINT('Ctrl Pts',(-6.79246102077101,-0.909925026569516,
2.37730584883283));
#10902=CARTESIAN_POINT('Ctrl Pts',(-6.22911235514946,-0.525814889228737,
2.40196226239673));
#10903=CARTESIAN_POINT('Ctrl Pts',(-6.07744456821118,0.138809074175696,
2.42661402385257));
#10904=CARTESIAN_POINT('Ctrl Pts',(-6.41824880300263,0.729027866722014,
2.45125992491537));
#10905=CARTESIAN_POINT('Ctrl Pts',(-7.06934122876124,0.929824149026898,
2.47589876067858));
#10906=CARTESIAN_POINT('Ctrl Pts',(-7.68299796183915,0.634246527935802,
2.50052933613646));
#10907=CARTESIAN_POINT('Ctrl Pts',(-7.93168967879738,0.000445263131447748,
2.52515045678013));
#10908=CARTESIAN_POINT('Ctrl Pts',(-7.68302213647328,-0.633094458923734,
2.54976094441856));
#10909=CARTESIAN_POINT('Ctrl Pts',(-7.07007700890629,-0.928102101680422,
2.57435962067245));
#10910=CARTESIAN_POINT('Ctrl Pts',(-6.42054771123064,-0.727833461900544,
2.59894532553828));
#10911=CARTESIAN_POINT('Ctrl Pts',(-6.08063030273252,-0.138905152375385,
2.62351690334527));
#10912=CARTESIAN_POINT('Ctrl Pts',(-6.20716604633801,0.411896009844242,
2.64398049630671));
#10913=CARTESIAN_POINT('Ctrl Pts',(-6.51199774209192,0.714676452673333,
2.66034317170459));
#10914=CARTESIAN_POINT('Ctrl Pts',(-6.80647130896726,0.843685013671235,
2.67261094147259));
#10915=CARTESIAN_POINT('Ctrl Pts',(-7.12812476587158,0.855502087711664,
2.68487433317324));
#10916=CARTESIAN_POINT('Ctrl Pts',(-7.43161948042588,0.749419002627999,
2.69713320958533));
#10917=CARTESIAN_POINT('Ctrl Pts',(-7.67521904640705,0.539636596661724,
2.7093874343511));
#10918=CARTESIAN_POINT('Ctrl Pts',(-7.82547325176268,0.255576344693996,
2.72163687040038));
#10919=CARTESIAN_POINT('Ctrl Pts',(-7.86123160253771,-0.0635635909156293,
2.73388138286896));
#10920=CARTESIAN_POINT('Ctrl Pts',(-7.76460027897753,-0.425533717492343,
2.74816074914963));
#10921=CARTESIAN_POINT('Ctrl Pts',(-7.47374360660769,-0.751894656156828,
2.76447137187111));
#10922=CARTESIAN_POINT('Ctrl Pts',(-7.00091436223893,-0.88782428734477,
2.78280870439184));
#10923=CARTESIAN_POINT('Ctrl Pts',(-6.52888862282209,-0.751805319722163,
2.80113347394993));
#10924=CARTESIAN_POINT('Ctrl Pts',(-6.2016684053735,-0.385612928895403,
2.81944525307317));
#10925=CARTESIAN_POINT('Ctrl Pts',(-6.11955382035284,0.0981170754742554,
2.83774361225262));
#10926=CARTESIAN_POINT('Ctrl Pts',(-6.30722625617569,0.551073055321834,
2.85602813457377));
#10927=CARTESIAN_POINT('Ctrl Pts',(-6.70680747045044,0.834525970819447,
2.87429840546262));
#10928=CARTESIAN_POINT('Ctrl Pts',(-7.19559869716282,0.861909407171868,
2.8925540164347));
#10929=CARTESIAN_POINT('Ctrl Pts',(-7.62360216624703,0.625277985438662,
2.91079457296321));
#10930=CARTESIAN_POINT('Ctrl Pts',(-7.86012925287909,0.197486531354187,
2.92901967711976));
#10931=CARTESIAN_POINT('Ctrl Pts',(-7.83237012712838,-0.289941720567784,
2.94722894753945));
#10932=CARTESIAN_POINT('Ctrl Pts',(-7.55008001741224,-0.687784692046307,
2.96542200407487));
#10933=CARTESIAN_POINT('Ctrl Pts',(-7.09977586824996,-0.874247976731781,
2.98359847915852));
#10934=CARTESIAN_POINT('Ctrl Pts',(-6.61974323779859,-0.792623075615972,
3.00175800933));
#10935=CARTESIAN_POINT('Ctrl Pts',(-6.257058130519,-0.468413543112272,3.0199002388146));
#10936=CARTESIAN_POINT('Ctrl Pts',(-6.12258713457564,-0.00138700255432796,
3.03802482606703));
#10937=CARTESIAN_POINT('Ctrl Pts',(-6.25706727378645,0.465139317147603,
3.05613142853581));
#10938=CARTESIAN_POINT('Ctrl Pts',(-6.61877666867083,0.788285032559405,
3.07421972093098));
#10939=CARTESIAN_POINT('Ctrl Pts',(-7.09647607914372,0.869376408975484,
3.09228937996591));
#10940=CARTESIAN_POINT('Ctrl Pts',(-7.54362920385282,0.68408153123717,3.11034009649877));
#10941=CARTESIAN_POINT('Ctrl Pts',(-7.82336210739947,0.28970919078182,3.12837156650594));
#10942=CARTESIAN_POINT('Ctrl Pts',(-7.85036951729978,-0.192518648808231,
3.1463834953635));
#10943=CARTESIAN_POINT('Ctrl Pts',(-7.61693284376151,-0.614735291409423,
3.16437560200786));
#10944=CARTESIAN_POINT('Ctrl Pts',(-7.19511476226595,-0.847778676228102,
3.18234760781168));
#10945=CARTESIAN_POINT('Ctrl Pts',(-6.7145098999882,-0.820710857786535,
3.20029925009486));
#10946=CARTESIAN_POINT('Ctrl Pts',(-6.32242256217712,-0.542413764760527,
3.21823027098919));
#10947=CARTESIAN_POINT('Ctrl Pts',(-6.13871066850024,-0.098686345015634,
3.23614042632575));
#10948=CARTESIAN_POINT('Ctrl Pts',(-6.21914065946509,0.374211025419683,
3.25402947870679));
#10949=CARTESIAN_POINT('Ctrl Pts',(-6.53845875539302,0.731406338297415,
3.27189720144838));
#10950=CARTESIAN_POINT('Ctrl Pts',(-6.99831755296742,0.863804065639348,
3.2897433804432));
#10951=CARTESIAN_POINT('Ctrl Pts',(-7.45757029965599,0.731409466469204,
3.30756780748229));
#10952=CARTESIAN_POINT('Ctrl Pts',(-7.77559982146972,0.37540881511312,3.32537028850097));
#10953=CARTESIAN_POINT('Ctrl Pts',(-7.85537931424834,-0.094642652826617,
3.34315063708933));
#10954=CARTESIAN_POINT('Ctrl Pts',(-7.67307624395954,-0.534539169893111,
3.36090867961867));
#10955=CARTESIAN_POINT('Ctrl Pts',(-7.28516805861167,-0.809670332991083,
3.37864425091963));
#10956=CARTESIAN_POINT('Ctrl Pts',(-6.81094328129299,-0.836216654728318,
3.39635719733567));
#10957=CARTESIAN_POINT('Ctrl Pts',(-6.39581795219668,-0.606687244699812,
3.41404737686194));
#10958=CARTESIAN_POINT('Ctrl Pts',(-6.16673282986248,-0.192016386472062,
3.43171465630725));
#10959=CARTESIAN_POINT('Ctrl Pts',(-6.19335105955753,0.280356102113162,
3.44935891493111));
#10960=CARTESIAN_POINT('Ctrl Pts',(-6.46683379484748,0.665660108445628,
3.46698004190314));
#10961=CARTESIAN_POINT('Ctrl Pts',(-6.90284795213186,0.846152102600437,
3.48457793824716));
#10962=CARTESIAN_POINT('Ctrl Pts',(-7.36737219772646,0.767129205800447,
3.50215251490095));
#10963=CARTESIAN_POINT('Ctrl Pts',(-7.71834143496065,0.453434200086869,
3.51970369457236));
#10964=CARTESIAN_POINT('Ctrl Pts',(-7.82645846631761,0.077080609195679,
3.53431012488451));
#10965=CARTESIAN_POINT('Ctrl Pts',(-7.78351602643939,-0.223766099777631,
3.54598350983127));
#10966=CARTESIAN_POINT('Ctrl Pts',(-7.65984666406284,-0.501195016191524,
3.55764904771478));
#10967=CARTESIAN_POINT('Ctrl Pts',(-7.36883520137935,-0.761421141511966,
3.57221624328425));
#10968=CARTESIAN_POINT('Ctrl Pts',(-6.90699782821215,-0.839986918687281,
3.58967328199228));
#10969=CARTESIAN_POINT('Ctrl Pts',(-6.5235772119384,-0.680444831465126,
3.60516965595896));
#10970=CARTESIAN_POINT('Ctrl Pts',(-6.29205860881578,-0.410854643842501,
3.6187136684483));
#10971=CARTESIAN_POINT('Ctrl Pts',(-6.19144251696091,-0.123792268925567,
3.63031232027941));
#10972=CARTESIAN_POINT('Ctrl Pts',(-6.20295651325157,0.179997595512823,
3.64190047202365));
#10973=CARTESIAN_POINT('Ctrl Pts',(-6.32432621115477,0.458374743512086,
3.65347812777622));
#10974=CARTESIAN_POINT('Ctrl Pts',(-6.53898438351643,0.672840241042802,
3.66504529364933));
#10975=CARTESIAN_POINT('Ctrl Pts',(-6.81680637706894,0.794134031701534,
3.67660197812095));
#10976=CARTESIAN_POINT('Ctrl Pts',(-7.11950248291682,0.805397533837699,
3.68814819174188));
#10977=CARTESIAN_POINT('Ctrl Pts',(-7.34163561569263,0.727628486768507,
3.69712044609008));
#10978=CARTESIAN_POINT('Ctrl Pts',(-7.53458281141515,0.599570945127131,
3.70608728556614));
#10979=CARTESIAN_POINT('Ctrl Pts',(-7.71503532521363,0.400461841999,3.71632891696956));
#10980=CARTESIAN_POINT('Ctrl Pts',(-7.82528743114405,0.0430926937144543,
3.73039630239659));
#10981=CARTESIAN_POINT('Ctrl Pts',(-7.74111169379658,-0.37323537543407,
3.74636272256909));
#10982=CARTESIAN_POINT('Ctrl Pts',(-7.44499573228645,-0.704767123835098,
3.76294659713056));
#10983=CARTESIAN_POINT('Ctrl Pts',(-7.00172600054551,-0.832350159693755,
3.78014508956006));
#10984=CARTESIAN_POINT('Ctrl Pts',(-6.55926311085665,-0.704755991680177,
3.79732045846001));
#10985=CARTESIAN_POINT('Ctrl Pts',(-6.2528315275211,-0.361772892660608,
3.81447281592693));
#10986=CARTESIAN_POINT('Ctrl Pts',(-6.17601189131465,0.0911409447444953,
3.83160228337755));
#10987=CARTESIAN_POINT('Ctrl Pts',(-6.35159897954253,0.514776986788965,
3.84870899394101));
#10988=CARTESIAN_POINT('Ctrl Pts',(-6.72535286944806,0.780122083208515,
3.86579309179979));
#10989=CARTESIAN_POINT('Ctrl Pts',(-7.13122870473182,0.802254155922275,
3.88095899359145));
#10990=CARTESIAN_POINT('Ctrl Pts',(-7.44985202071078,0.662844517922881,
3.89421470788503));
#10991=CARTESIAN_POINT('Ctrl Pts',(-7.66049480984587,0.452421922662202,
3.90556689264628));
#10992=CARTESIAN_POINT('Ctrl Pts',(-7.77936222711058,0.179641079514188,
3.91690927461427));
#10993=CARTESIAN_POINT('Ctrl Pts',(-7.79055864897702,-0.117447939280878,
3.92824190893221));
#10994=CARTESIAN_POINT('Ctrl Pts',(-7.69235883457516,-0.397692735498425,
3.93956485365948));
#10995=CARTESIAN_POINT('Ctrl Pts',(-7.4988193112063,-0.622862064421365,
3.95087816922642));
#10996=CARTESIAN_POINT('Ctrl Pts',(-7.23669309425985,-0.760857052520071,
3.96218191668704));
#10997=CARTESIAN_POINT('Ctrl Pts',(-6.84397122474983,-0.806385392143749,
3.97724090685452));
#10998=CARTESIAN_POINT('Ctrl Pts',(-6.3759149329141,-0.581575494059258,
3.99604104936904));
#10999=CARTESIAN_POINT('Ctrl Pts',(-6.14801487092373,-0.00140577011587543,
4.01856401164168));
#11000=CARTESIAN_POINT('Ctrl Pts',(-6.37569406553146,0.577216837917985,
4.04105035155356));
#11001=CARTESIAN_POINT('Ctrl Pts',(-6.93503804704956,0.846504117962824,
4.06350067666592));
#11002=CARTESIAN_POINT('Ctrl Pts',(-7.52735353249786,0.663517124905538,
4.08591563261074));
#11003=CARTESIAN_POINT('Ctrl Pts',(-7.83667549320556,0.127633503183688,
4.10829588960443));
#11004=CARTESIAN_POINT('Ctrl Pts',(-7.69892862810743,-0.475216209100622,
4.13064214875721));
#11005=CARTESIAN_POINT('Ctrl Pts',(-7.24587822138796,-0.783213519985818,
4.15047591997482));
#11006=CARTESIAN_POINT('Ctrl Pts',(-6.78448909503242,-0.770150049272615,
4.16780939837816));
#11007=CARTESIAN_POINT('Ctrl Pts',(-6.44291255401028,-0.573358437418835,
4.18265244830762));
#11008=CARTESIAN_POINT('Ctrl Pts',(-6.23727444607057,-0.236582538920206,
4.19748151807985));
#11009=CARTESIAN_POINT('Ctrl Pts',(-6.21750233201011,0.156779347523281,
4.21229685032696));
#11010=CARTESIAN_POINT('Ctrl Pts',(-6.38851989967645,0.511421035774412,
4.22709868951428));
#11011=CARTESIAN_POINT('Ctrl Pts',(-6.68127276436824,0.721655369840554,
4.24065490665371));
#11012=CARTESIAN_POINT('Ctrl Pts',(-6.99873870462004,0.781500222137114,
4.25296927229394));
#11013=CARTESIAN_POINT('Ctrl Pts',(-7.28423799128053,0.727580241858167,
4.26404501085876));
#11014=CARTESIAN_POINT('Ctrl Pts',(-7.52996735384668,0.573044604556925,
4.27511366794562));
#11015=CARTESIAN_POINT('Ctrl Pts',(-7.70249233600175,0.339504000304913,
4.28617535676904));
#11016=CARTESIAN_POINT('Ctrl Pts',(-7.77704029199075,0.0596812865399207,
4.29723019232866));
#11017=CARTESIAN_POINT('Ctrl Pts',(-7.73493077249201,-0.32516426809182,
4.31196099263524));
#11018=CARTESIAN_POINT('Ctrl Pts',(-7.48195320169677,-0.642258532616097,
4.32667855077855));
#11019=CARTESIAN_POINT('Ctrl Pts',(-7.11676447072565,-0.768672906025829,
4.34138335007881));
#11020=CARTESIAN_POINT('Ctrl Pts',(-6.82822052968084,-0.75826459078673,
4.35240569057047));
#11021=CARTESIAN_POINT('Ctrl Pts',(-6.56324655367934,-0.642480501470498,
4.36342189483669));
#11022=CARTESIAN_POINT('Ctrl Pts',(-6.3590246126422,-0.438361948172784,
4.37443208856579));
#11023=CARTESIAN_POINT('Ctrl Pts',(-6.24366823031993,-0.173725992278803,
4.38543639651659));
#11024=CARTESIAN_POINT('Ctrl Pts',(-6.23278862096309,0.114603786226641,
4.39643494391794));
#11025=CARTESIAN_POINT('Ctrl Pts',(-6.32818140570146,0.3866727001158,4.40742785948479));
#11026=CARTESIAN_POINT('Ctrl Pts',(-6.54732728408833,0.641795528726263,
4.42024651101618));
#11027=CARTESIAN_POINT('Ctrl Pts',(-6.90966296029133,0.792450205988824,
4.43488744119146));
#11028=CARTESIAN_POINT('Ctrl Pts',(-7.34497884959273,0.718229352606656,
4.45134684847234));
#11029=CARTESIAN_POINT('Ctrl Pts',(-7.67373744220819,0.42439860304808,4.46779506017063));
#11030=CARTESIAN_POINT('Ctrl Pts',(-7.7957623026863,0.000795392209376382,
4.48423253597012));
#11031=CARTESIAN_POINT('Ctrl Pts',(-7.6737681501059,-0.422451523433032,
4.50065973137187));
#11032=CARTESIAN_POINT('Ctrl Pts',(-7.34550270887416,-0.715780174479536,
4.51707711746896));
#11033=CARTESIAN_POINT('Ctrl Pts',(-6.91173568096419,-0.789442989854855,
4.53348515869499));
#11034=CARTESIAN_POINT('Ctrl Pts',(-6.50548543634235,-0.62113576023861,
4.54988433137086));
#11035=CARTESIAN_POINT('Ctrl Pts',(-6.25117725190974,-0.26266942709969,
4.56627511486019));
#11036=CARTESIAN_POINT('Ctrl Pts',(-6.22657268391725,0.175941615799059,
4.58265798957595));
#11037=CARTESIAN_POINT('Ctrl Pts',(-6.43900037753832,0.560237327905976,
4.59903344336352));
#11038=CARTESIAN_POINT('Ctrl Pts',(-6.82315231070266,0.772532064615231,
4.61540196293227));
#11039=CARTESIAN_POINT('Ctrl Pts',(-7.2612181287951,0.747894614274433,4.63176404577646));
#11040=CARTESIAN_POINT('Ctrl Pts',(-7.61885424416052,0.494109349486934,
4.64812018315545));
#11041=CARTESIAN_POINT('Ctrl Pts',(-7.78669901230814,0.0889725746862699,
4.66447087596232));
#11042=CARTESIAN_POINT('Ctrl Pts',(-7.72532501848925,-0.270994143806812,
4.67809233336064));
#11043=CARTESIAN_POINT('Ctrl Pts',(-7.56738721688822,-0.506594326857297,
4.68898728035258));
#11044=CARTESIAN_POINT('Ctrl Pts',(-7.35097564028756,-0.689891456361417,
4.69988083117445));
#11045=CARTESIAN_POINT('Ctrl Pts',(-7.0003169174225,-0.79110738140522,4.71349530909451));
#11046=CARTESIAN_POINT('Ctrl Pts',(-6.57937611771461,-0.669773743535281,
4.72982925479887));
#11047=CARTESIAN_POINT('Ctrl Pts',(-6.28761734218788,-0.343284450620702,
4.74616028288309));
#11048=CARTESIAN_POINT('Ctrl Pts',(-6.21426971041073,0.0883871334668474,
4.76248890194073));
#11049=CARTESIAN_POINT('Ctrl Pts',(-6.38182100128212,0.492840639406237,
4.77881561989744));
#11050=CARTESIAN_POINT('Ctrl Pts',(-6.73884045313308,0.746153973023737,
4.79514095601288));
#11051=CARTESIAN_POINT('Ctrl Pts',(-7.17589338359863,0.770679755263529,
4.81146540426486));
#11052=CARTESIAN_POINT('Ctrl Pts',(-7.55900114520461,0.55894423669953,4.82778951061359));
#11053=CARTESIAN_POINT('Ctrl Pts',(-7.77075750409873,0.175788412965931,
4.84411370102291));
#11054=CARTESIAN_POINT('Ctrl Pts',(-7.74620736592161,-0.261233995076225,
4.86043866853608));
#11055=CARTESIAN_POINT('Ctrl Pts',(-7.49294321470503,-0.618448872812403,
4.87676449790797));
#11056=CARTESIAN_POINT('Ctrl Pts',(-7.08837163954946,-0.785730122461179,
4.89309260172666));
#11057=CARTESIAN_POINT('Ctrl Pts',(-6.65674407499508,-0.712671607108413,
4.90942182102584));
#11058=CARTESIAN_POINT('Ctrl Pts',(-6.33017289353631,-0.420518596063947,
4.92575590410514));
#11059=CARTESIAN_POINT('Ctrl Pts',(-6.2493887150478,-0.140566474730618,
4.93664355063335));
#11060=CARTESIAN_POINT('Ctrl Pts',(-6.24936976727053,0.000312488344807942,
4.94209250793942));
#11061=CARTESIAN_POINT('Ctrl Pts',(-6.21496022479178,0.00193045739649654,
1.00003735833913));
#11062=CARTESIAN_POINT('Ctrl Pts',(-6.21498003690632,0.149236475283263,
1.0057349030646));
#11063=CARTESIAN_POINT('Ctrl Pts',(-6.29946146307499,0.442287265692152,
1.01713084057243));
#11064=CARTESIAN_POINT('Ctrl Pts',(-6.64173420840598,0.74861847420515,1.03425315186381));
#11065=CARTESIAN_POINT('Ctrl Pts',(-7.09490182459049,0.825432047669671,
1.05139783360786));
#11066=CARTESIAN_POINT('Ctrl Pts',(-7.52036826388768,0.649617795679984,
1.06856728953495));
#11067=CARTESIAN_POINT('Ctrl Pts',(-7.7871742517923,0.273479603576055,1.08576001517786));
#11068=CARTESIAN_POINT('Ctrl Pts',(-7.81315997530967,-0.187447249693266,
1.10297754661545));
#11069=CARTESIAN_POINT('Ctrl Pts',(-7.589586767382,-0.592199963068705,1.12021926119168));
#11070=CARTESIAN_POINT('Ctrl Pts',(-7.18437407174804,-0.816243588302344,
1.13748556186172));
#11071=CARTESIAN_POINT('Ctrl Pts',(-6.72148059457952,-0.790355142963932,
1.15477626219657));
#11072=CARTESIAN_POINT('Ctrl Pts',(-6.34262910012066,-0.52172948451145,
1.17209170042211));
#11073=CARTESIAN_POINT('Ctrl Pts',(-6.19449971679954,-0.163784023548138,
1.18654139527825));
#11074=CARTESIAN_POINT('Ctrl Pts',(-6.2033859162291,0.137380889459928,1.19811412071467));
#11075=CARTESIAN_POINT('Ctrl Pts',(-6.29449904481813,0.424787607736377,
1.20969506869488));
#11076=CARTESIAN_POINT('Ctrl Pts',(-6.55315191262231,0.714650845840973,
1.22418580731435));
#11077=CARTESIAN_POINT('Ctrl Pts',(-7.0019550394566,0.843993903272686,1.24159980818703));
#11078=CARTESIAN_POINT('Ctrl Pts',(-7.45128651383865,0.714642167033589,
1.25903832129017));
#11079=CARTESIAN_POINT('Ctrl Pts',(-7.76342536249333,0.365519355718316,
1.27650157939527));
#11080=CARTESIAN_POINT('Ctrl Pts',(-7.84206012434238,-0.0967940191462743,
1.29398943844924));
#11081=CARTESIAN_POINT('Ctrl Pts',(-7.66243479502456,-0.530701874726786,
1.311501908922));
#11082=CARTESIAN_POINT('Ctrl Pts',(-7.27894550868061,-0.802913947461582,
1.3290389166792));
#11083=CARTESIAN_POINT('Ctrl Pts',(-6.80875585148875,-0.829412645711587,
1.34660041024838));
#11084=CARTESIAN_POINT('Ctrl Pts',(-6.39596178700798,-0.601376268456168,
1.3641863119731));
#11085=CARTESIAN_POINT('Ctrl Pts',(-6.16744602527253,-0.18810074316643,
1.38179653848221));
#11086=CARTESIAN_POINT('Ctrl Pts',(-6.19386832849657,0.284055727066803,
1.39943099486938));
#11087=CARTESIAN_POINT('Ctrl Pts',(-6.46781735673514,0.670315409844122,
1.41708956636422));
#11088=CARTESIAN_POINT('Ctrl Pts',(-6.905874703008,0.851860949298453,1.43477214942586));
#11089=CARTESIAN_POINT('Ctrl Pts',(-7.37400527438391,0.772425993272578,
1.45247857106921));
#11090=CARTESIAN_POINT('Ctrl Pts',(-7.72859756382396,0.455648564419921,
1.47020877245192));
#11091=CARTESIAN_POINT('Ctrl Pts',(-7.86046618774004,-0.00176530696331421,
1.4879623972667));
#11092=CARTESIAN_POINT('Ctrl Pts',(-7.72860440581187,-0.459992961560558,
1.50573970438362));
#11093=CARTESIAN_POINT('Ctrl Pts',(-7.43196756428821,-0.724892207153614,
1.52057285972636));
#11094=CARTESIAN_POINT('Ctrl Pts',(-7.13716670831516,-0.818376347595012,
1.53245209596733));
#11095=CARTESIAN_POINT('Ctrl Pts',(-6.82779061711728,-0.827560724830197,
1.54433902667896));
#11096=CARTESIAN_POINT('Ctrl Pts',(-6.47583393331273,-0.681911359548126,
1.55854925722825));
#11097=CARTESIAN_POINT('Ctrl Pts',(-6.21016594208147,-0.330954869083988,
1.57509380975784));
#11098=CARTESIAN_POINT('Ctrl Pts',(-6.14705675793353,0.0870687063999194,
1.59099390692264));
#11099=CARTESIAN_POINT('Ctrl Pts',(-6.29178381216594,0.484946937091849,
1.60691177329472));
#11100=CARTESIAN_POINT('Ctrl Pts',(-6.60953147959695,0.765383168267148,
1.62284694312522));
#11101=CARTESIAN_POINT('Ctrl Pts',(-7.02306130867876,0.859862600782519,
1.63879940878992));
#11102=CARTESIAN_POINT('Ctrl Pts',(-7.43209092835715,0.744843356641513,
1.65476878917197));
#11103=CARTESIAN_POINT('Ctrl Pts',(-7.7360822935237,0.448060979198733,1.67075513675566));
#11104=CARTESIAN_POINT('Ctrl Pts',(-7.87645764778973,-0.00385954133554831,
1.6885372052021));
#11105=CARTESIAN_POINT('Ctrl Pts',(-7.72834851689841,-0.516119382107579,
1.70812061510533));
#11106=CARTESIAN_POINT('Ctrl Pts',(-7.25468100412709,-0.856808986327443,
1.7295133131787));
#11107=CARTESIAN_POINT('Ctrl Pts',(-6.72053536605562,-0.834270555713778,
1.7491497241697));
#11108=CARTESIAN_POINT('Ctrl Pts',(-6.33474611188452,-0.555924840423259,
1.76701999702058));
#11109=CARTESIAN_POINT('Ctrl Pts',(-6.14885811639311,-0.170590221039593,
1.78311889654665));
#11110=CARTESIAN_POINT('Ctrl Pts',(-6.17018600999163,0.25761300576502,1.79923302183049));
#11111=CARTESIAN_POINT('Ctrl Pts',(-6.3938333344896,0.623621296817837,1.81536201710917));
#11112=CARTESIAN_POINT('Ctrl Pts',(-6.76559988585565,0.838322726739336,
1.83150595091894));
#11113=CARTESIAN_POINT('Ctrl Pts',(-7.19533204419046,0.849214134207467,
1.8476636842115));
#11114=CARTESIAN_POINT('Ctrl Pts',(-7.51408506059226,0.685479419534324,
1.86114130347342));
#11115=CARTESIAN_POINT('Ctrl Pts',(-7.69935073706812,0.475097794954268,
1.87193087421034));
#11116=CARTESIAN_POINT('Ctrl Pts',(-7.82756719690158,0.225696299951463,
1.88272501062167));
#11117=CARTESIAN_POINT('Ctrl Pts',(-7.86345218589821,-0.131510401233362,
1.8962239903695));
#11118=CARTESIAN_POINT('Ctrl Pts',(-7.69613807595462,-0.528918375423483,
1.91243912933416));
#11119=CARTESIAN_POINT('Ctrl Pts',(-7.35867518420911,-0.798157754455865,
1.9286640042301));
#11120=CARTESIAN_POINT('Ctrl Pts',(-6.96881533719357,-0.86658287393614,
1.94355059132535));
#11121=CARTESIAN_POINT('Ctrl Pts',(-6.62565014145497,-0.774407287161083,
1.95709390795204));
#11122=CARTESIAN_POINT('Ctrl Pts',(-6.36815349730449,-0.584571010932259,
1.96928914184098));
#11123=CARTESIAN_POINT('Ctrl Pts',(-6.19791761268333,-0.313459785840694,
1.9814915020885));
#11124=CARTESIAN_POINT('Ctrl Pts',(-6.13824564444744,0.00126222564801271,
1.99370039068808));
#11125=CARTESIAN_POINT('Ctrl Pts',(-6.19791470426975,0.316044722401465,
2.00591590248117));
#11126=CARTESIAN_POINT('Ctrl Pts',(-6.36840364468326,0.587805810914203,
2.01813791913327));
#11127=CARTESIAN_POINT('Ctrl Pts',(-6.62655450559938,0.777726269115704,
2.03036614812532));
#11128=CARTESIAN_POINT('Ctrl Pts',(-7.03995270037433,0.890005270964902,
2.04667918548612));
#11129=CARTESIAN_POINT('Ctrl Pts',(-7.57875104075548,0.724669890533431,
2.06708353353878));
#11130=CARTESIAN_POINT('Ctrl Pts',(-7.91803573835962,0.137269411407317,
2.09159331225351));
#11131=CARTESIAN_POINT('Ctrl Pts',(-7.76706117168378,-0.52400406240848,
2.1161247857463));
#11132=CARTESIAN_POINT('Ctrl Pts',(-7.20611421556751,-0.906687379904759,
2.14067751861688));
#11133=CARTESIAN_POINT('Ctrl Pts',(-6.53407310359242,-0.805456679357255,
2.16525004772343));
#11134=CARTESIAN_POINT('Ctrl Pts',(-6.10996474228539,-0.273794595356463,
2.18984134725865));
#11135=CARTESIAN_POINT('Ctrl Pts',(-6.16073373652603,0.404915665396,2.21445019333614));
#11136=CARTESIAN_POINT('Ctrl Pts',(-6.65992496701694,0.868206142671759,
2.23907543071713));
#11137=CARTESIAN_POINT('Ctrl Pts',(-7.34139465906004,0.868284001000674,
2.26371586031783));
#11138=CARTESIAN_POINT('Ctrl Pts',(-7.84127886499866,0.404554221629114,
2.28837028439299));
#11139=CARTESIAN_POINT('Ctrl Pts',(-7.89232330647337,-0.275743068898642,
2.31303748987548));
#11140=CARTESIAN_POINT('Ctrl Pts',(-7.46681769389894,-0.809401324879221,
2.33771625419332));
#11141=CARTESIAN_POINT('Ctrl Pts',(-6.79163727905948,-0.911218932362134,
2.36240534623989));
#11142=CARTESIAN_POINT('Ctrl Pts',(-6.22723819401461,-0.526470972456904,
2.38710352441179));
#11143=CARTESIAN_POINT('Ctrl Pts',(-6.07515776140191,0.139671239855932,
2.41180954160707));
#11144=CARTESIAN_POINT('Ctrl Pts',(-6.4168642269915,0.731580916682001,2.43652214117368));
#11145=CARTESIAN_POINT('Ctrl Pts',(-7.07009497004517,0.933103386959657,
2.46124006421744));
#11146=CARTESIAN_POINT('Ctrl Pts',(-7.6861192958364,0.63645551279314,2.48596203741659));
#11147=CARTESIAN_POINT('Ctrl Pts',(-7.93594161987389,-5.53991550515054E-5,
2.51068680546929));
#11148=CARTESIAN_POINT('Ctrl Pts',(-7.68613683601064,-0.636663310280273,
2.53541304689358));
#11149=CARTESIAN_POINT('Ctrl Pts',(-7.06997132216139,-0.933290058159735,
2.56013958420914));
#11150=CARTESIAN_POINT('Ctrl Pts',(-6.41666529744918,-0.731923724485437,
2.58486487069508));
#11151=CARTESIAN_POINT('Ctrl Pts',(-6.07456382672486,-0.139335588546712,
2.60958819020872));
#11152=CARTESIAN_POINT('Ctrl Pts',(-6.20189998741875,0.415187630242587,
2.63018704219427));
#11153=CARTESIAN_POINT('Ctrl Pts',(-6.50889656590471,0.720128182080066,
2.64666510151446));
#11154=CARTESIAN_POINT('Ctrl Pts',(-6.80552668601887,0.850092546186389,
2.65902201878275));
#11155=CARTESIAN_POINT('Ctrl Pts',(-7.12961665841912,0.862002494205028,
2.6713774719234));
#11156=CARTESIAN_POINT('Ctrl Pts',(-7.43548347744342,0.755101152634445,
2.68373125908594));
#11157=CARTESIAN_POINT('Ctrl Pts',(-7.68104236213469,0.543633793008857,
2.69608312748103));
#11158=CARTESIAN_POINT('Ctrl Pts',(-7.83254697985538,0.257228154096008,
2.70843323313999));
#11159=CARTESIAN_POINT('Ctrl Pts',(-7.86861092865602,-0.0646242885083314,
2.72078087920498));
#11160=CARTESIAN_POINT('Ctrl Pts',(-7.77114357730519,-0.429760638880875,
2.73518461873645));
#11161=CARTESIAN_POINT('Ctrl Pts',(-7.47768041418785,-0.759071075031029,
2.75164059738));
#11162=CARTESIAN_POINT('Ctrl Pts',(-7.00044547067498,-0.896286834016264,
2.77014692551625));
#11163=CARTESIAN_POINT('Ctrl Pts',(-6.52384755468618,-0.758970388215617,
2.78864723612747));
#11164=CARTESIAN_POINT('Ctrl Pts',(-6.19334012335843,-0.38912725030458,
2.80714040083053));
#11165=CARTESIAN_POINT('Ctrl Pts',(-6.1103571328977,0.0995956644790968,
2.82562612963652));
#11166=CARTESIAN_POINT('Ctrl Pts',(-6.30000871896293,0.557383043092008,
2.84410374158365));
#11167=CARTESIAN_POINT('Ctrl Pts',(-6.70395782539939,0.843960256355834,
2.86257284280838));
#11168=CARTESIAN_POINT('Ctrl Pts',(-7.1982573895186,0.871674220369247,2.88103270749344));
#11169=CARTESIAN_POINT('Ctrl Pts',(-7.63122519892655,0.632319691352436,
2.89948325375147));
#11170=CARTESIAN_POINT('Ctrl Pts',(-7.87057865226024,0.199460779002233,
2.91792304408701));
#11171=CARTESIAN_POINT('Ctrl Pts',(-7.84249835142399,-0.293910837809749,
2.93635365094154));
#11172=CARTESIAN_POINT('Ctrl Pts',(-7.55670690192362,-0.696723750004534,
2.95477217425725));
#11173=CARTESIAN_POINT('Ctrl Pts',(-7.10066709958465,-0.885581860171592,
2.97317926541403));
#11174=CARTESIAN_POINT('Ctrl Pts',(-6.61437502277845,-0.802910390411064,
2.99157433709339));
#11175=CARTESIAN_POINT('Ctrl Pts',(-6.24685080367674,-0.474398196000392,
3.00995694611218));
#11176=CARTESIAN_POINT('Ctrl Pts',(-6.11053734543688,-0.00103335347657871,
3.02832662126797));
#11177=CARTESIAN_POINT('Ctrl Pts',(-6.24686361423024,0.471957306655142,
3.04668290533691));
#11178=CARTESIAN_POINT('Ctrl Pts',(-6.61366423072175,0.799673263093506,
3.06502535163926));
#11179=CARTESIAN_POINT('Ctrl Pts',(-7.09821994184268,0.881944668383278,
3.08335351554756));
#11180=CARTESIAN_POINT('Ctrl Pts',(-7.55190977568874,0.693957832127035,
3.10166696504459));
#11181=CARTESIAN_POINT('Ctrl Pts',(-7.83580785554474,0.293739343295185,
3.11996527109821));
#11182=CARTESIAN_POINT('Ctrl Pts',(-7.86323708904419,-0.195759930573144,
3.13824801170802));
#11183=CARTESIAN_POINT('Ctrl Pts',(-7.62623911633122,-0.624446980074989,
3.15651477910607));
#11184=CARTESIAN_POINT('Ctrl Pts',(-7.19787659404976,-0.861121517451799,
3.17476516277629));
#11185=CARTESIAN_POINT('Ctrl Pts',(-6.70970363928432,-0.83364058160835,
3.19299876958912));
#11186=CARTESIAN_POINT('Ctrl Pts',(-6.31135370706244,-0.550913868799662,
3.21121520727279));
#11187=CARTESIAN_POINT('Ctrl Pts',(-6.12466269110821,-0.100022524381656,
3.22941409750615));
#11188=CARTESIAN_POINT('Ctrl Pts',(-6.20639624300564,0.380608586344866,
3.24759506582347));
#11189=CARTESIAN_POINT('Ctrl Pts',(-6.53098669794507,0.743718343207315,
3.26575774696197));
#11190=CARTESIAN_POINT('Ctrl Pts',(-6.99853026788513,0.878339630134887,
3.28390178877985));
#11191=CARTESIAN_POINT('Ctrl Pts',(-7.46554282551143,0.743718514945607,
3.30202684061782));
#11192=CARTESIAN_POINT('Ctrl Pts',(-7.78900382487124,0.381652261179626,
3.32013256737826));
#11193=CARTESIAN_POINT('Ctrl Pts',(-7.87016557654628,-0.0964892509804086,
3.33821863849062));
#11194=CARTESIAN_POINT('Ctrl Pts',(-7.68470472929137,-0.544027709032238,
3.35628473667664));
#11195=CARTESIAN_POINT('Ctrl Pts',(-7.29000983952638,-0.823982249810174,
3.3743305505273));
#11196=CARTESIAN_POINT('Ctrl Pts',(-6.80741892018219,-0.851004345886966,
3.39235577973309));
#11197=CARTESIAN_POINT('Ctrl Pts',(-6.38491355915793,-0.617402275389218,
3.41036013559038));
#11198=CARTESIAN_POINT('Ctrl Pts',(-6.15172476360541,-0.195316421174017,
3.42834333636049));
#11199=CARTESIAN_POINT('Ctrl Pts',(-6.17881634954805,0.285559220418923,
3.44630511117001));
#11200=CARTESIAN_POINT('Ctrl Pts',(-6.45724574362916,0.677841532703307,
3.4642452037166));
#11201=CARTESIAN_POINT('Ctrl Pts',(-6.90119282927497,0.861622534318975,
3.48216335628587));
#11202=CARTESIAN_POINT('Ctrl Pts',(-7.37421145008331,0.781158702191044,
3.50005935104225));
#11203=CARTESIAN_POINT('Ctrl Pts',(-7.73162808926433,0.461706158499515,
3.51793291265731));
#11204=CARTESIAN_POINT('Ctrl Pts',(-7.84174018381471,0.0784155713339669,
3.53280876811356));
#11205=CARTESIAN_POINT('Ctrl Pts',(-7.79800443241366,-0.227989827411191,
3.54469790503734));
#11206=CARTESIAN_POINT('Ctrl Pts',(-7.67204661082408,-0.51055230958309,
3.55657940142524));
#11207=CARTESIAN_POINT('Ctrl Pts',(-7.37563777804564,-0.775605435513216,
3.57141711961568));
#11208=CARTESIAN_POINT('Ctrl Pts',(-6.90521308169463,-0.855631913255045,
3.58919913713307));
#11209=CARTESIAN_POINT('Ctrl Pts',(-6.51465060638591,-0.69311751818218,
3.60498452681796));
#11210=CARTESIAN_POINT('Ctrl Pts',(-6.27881507231595,-0.418500796234524,
3.61878116804605));
#11211=CARTESIAN_POINT('Ctrl Pts',(-6.17632312766382,-0.126080287612221,
3.63059654719756));
#11212=CARTESIAN_POINT('Ctrl Pts',(-6.18805220951868,0.183382360639241,
3.64240124248303));
#11213=CARTESIAN_POINT('Ctrl Pts',(-6.31169162966109,0.466959088490852,
3.65419545058532));
#11214=CARTESIAN_POINT('Ctrl Pts',(-6.53036023200659,0.685431933329652,
3.66597892390944));
#11215=CARTESIAN_POINT('Ctrl Pts',(-6.81337429752307,0.808990321171382,
3.67775183119918));
#11216=CARTESIAN_POINT('Ctrl Pts',(-7.12172107959111,0.820464843886967,
3.68951368947386));
#11217=CARTESIAN_POINT('Ctrl Pts',(-7.34800121451071,0.741243120114073,
3.69865368566005));
#11218=CARTESIAN_POINT('Ctrl Pts',(-7.54454733227601,0.610797496612732,
3.70778790363217));
#11219=CARTESIAN_POINT('Ctrl Pts',(-7.72836238347323,0.407977213954234,
3.71822051453867));
#11220=CARTESIAN_POINT('Ctrl Pts',(-7.84066640889921,0.0439535641028487,
3.73255015514311));
#11221=CARTESIAN_POINT('Ctrl Pts',(-7.75492245715288,-0.38011715810829,
3.74881430963631));
#11222=CARTESIAN_POINT('Ctrl Pts',(-7.45331040205047,-0.717798573300966,
3.76570679042953));
#11223=CARTESIAN_POINT('Ctrl Pts',(-7.00184044230431,-0.847738465434875,
3.78322435324808));
#11224=CARTESIAN_POINT('Ctrl Pts',(-6.55122324812836,-0.717788116639949,
3.80071732111976));
#11225=CARTESIAN_POINT('Ctrl Pts',(-6.23916998145882,-0.368503730982292,
3.81818563971551));
#11226=CARTESIAN_POINT('Ctrl Pts',(-6.16095439337113,0.0926910769171822,
3.83562938690738));
#11227=CARTESIAN_POINT('Ctrl Pts',(-6.33974396233009,0.524030742822703,
3.8530484228516));
#11228=CARTESIAN_POINT('Ctrl Pts',(-6.72027090623596,0.794170891984653,
3.8704431308788));
#11229=CARTESIAN_POINT('Ctrl Pts',(-7.1334479191549,0.816691600475571,3.88588284353928));
#11230=CARTESIAN_POINT('Ctrl Pts',(-7.457766743847,0.67478730266217,3.89937585423884));
#11231=CARTESIAN_POINT('Ctrl Pts',(-7.67215648924734,0.46061316986074,3.91093083109438));
#11232=CARTESIAN_POINT('Ctrl Pts',(-7.79312888962497,0.182997472536088,
3.92247465031486));
#11233=CARTESIAN_POINT('Ctrl Pts',(-7.80451620006278,-0.119330813613606,
3.93400773053184));
#11234=CARTESIAN_POINT('Ctrl Pts',(-7.70459309568693,-0.404491448730027,
3.94552981955708));
#11235=CARTESIAN_POINT('Ctrl Pts',(-7.50767277094898,-0.633584373326835,
3.95704107739786));
#11236=CARTESIAN_POINT('Ctrl Pts',(-7.24100086035615,-0.773972195308569,
3.96854144986818));
#11237=CARTESIAN_POINT('Ctrl Pts',(-6.84150953053856,-0.820277435822203,
3.98386071903549));
#11238=CARTESIAN_POINT('Ctrl Pts',(-6.3654633640183,-0.591611081989893,
4.00298376177583));
#11239=CARTESIAN_POINT('Ctrl Pts',(-6.1337576390178,-0.00166122908455176,
4.02588709218193));
#11240=CARTESIAN_POINT('Ctrl Pts',(-6.36524032244932,0.586552139022073,
4.0487488089353));
#11241=CARTESIAN_POINT('Ctrl Pts',(-6.93373182771633,0.860206205841142,
4.07156736576551));
#11242=CARTESIAN_POINT('Ctrl Pts',(-7.53554145104219,0.674250442998106,
4.0943439987415));
#11243=CARTESIAN_POINT('Ctrl Pts',(-7.84970605920547,0.129907369813062,
4.11707862258703));
#11244=CARTESIAN_POINT('Ctrl Pts',(-7.70979429430066,-0.482242979932142,
4.13977201588358));
#11245=CARTESIAN_POINT('Ctrl Pts',(-7.24987944831994,-0.794866937844285,
4.1599071059334));
#11246=CARTESIAN_POINT('Ctrl Pts',(-6.78164215790337,-0.78159338937728,
4.17749998328314));
#11247=CARTESIAN_POINT('Ctrl Pts',(-6.43508142553994,-0.581914508121684,
4.19256186736058));
#11248=CARTESIAN_POINT('Ctrl Pts',(-6.22649440794211,-0.240291343540091,
4.20760570805015));
#11249=CARTESIAN_POINT('Ctrl Pts',(-6.20646282732663,0.158625568218903,
4.22263173846367));
#11250=CARTESIAN_POINT('Ctrl Pts',(-6.37985866256235,0.518181945746219,
4.23763986606553));
#11251=CARTESIAN_POINT('Ctrl Pts',(-6.676621959726,0.731271387526176,4.25138360802136));
#11252=CARTESIAN_POINT('Ctrl Pts',(-6.99833352149209,0.791913885519912,
4.26386326383385));
#11253=CARTESIAN_POINT('Ctrl Pts',(-7.28759771419049,0.737272473718823,
4.27508616182068));
#11254=CARTESIAN_POINT('Ctrl Pts',(-7.53651652643787,0.580727616932713,
4.2862994040904));
#11255=CARTESIAN_POINT('Ctrl Pts',(-7.71123812831514,0.344194682380573,
4.29750342874701));
#11256=CARTESIAN_POINT('Ctrl Pts',(-7.78672009233439,0.0608522761698529,
4.3086983822003));
#11257=CARTESIAN_POINT('Ctrl Pts',(-7.74407670626882,-0.328749819328367,
4.32361209918105));
#11258=CARTESIAN_POINT('Ctrl Pts',(-7.488016071979,-0.649656030398014,4.33851040798963));
#11259=CARTESIAN_POINT('Ctrl Pts',(-7.11855150721405,-0.77754314811613,
4.35338822144775));
#11260=CARTESIAN_POINT('Ctrl Pts',(-6.82669090383297,-0.767006673780784,
4.36453838462225));
#11261=CARTESIAN_POINT('Ctrl Pts',(-6.55873239018928,-0.649916384419054,
4.37567961202239));
#11262=CARTESIAN_POINT('Ctrl Pts',(-6.35226305448287,-0.443537303631106,
4.38681229399512));
#11263=CARTESIAN_POINT('Ctrl Pts',(-6.23566062987361,-0.176041345419126,
4.39793651633846));
#11264=CARTESIAN_POINT('Ctrl Pts',(-6.22467492822247,0.115336230842568,
4.40905210574612));
#11265=CARTESIAN_POINT('Ctrl Pts',(-6.32105446110734,0.390215990371737,
4.42015973648825));
#11266=CARTESIAN_POINT('Ctrl Pts',(-6.54241539602128,0.647903422644043,
4.4331081071576));
#11267=CARTESIAN_POINT('Ctrl Pts',(-6.90830837563262,0.800018879819483,
4.44789438520924));
#11268=CARTESIAN_POINT('Ctrl Pts',(-7.34773390300693,0.725076966311309,
4.46451191698296));
#11269=CARTESIAN_POINT('Ctrl Pts',(-7.67945563591345,0.428569859702225,
4.48111131802776));
#11270=CARTESIAN_POINT('Ctrl Pts',(-7.8025196238951,0.00128543290513052,
4.49769375395874));
#11271=CARTESIAN_POINT('Ctrl Pts',(-7.67949177727457,-0.425464330000851,
4.51425934408901));
#11272=CARTESIAN_POINT('Ctrl Pts',(-7.34861601444808,-0.721093459242237,
4.5308086687758));
#11273=CARTESIAN_POINT('Ctrl Pts',(-6.91158610847141,-0.795285145135524,
4.54734208939356));
#11274=CARTESIAN_POINT('Ctrl Pts',(-6.50245425438708,-0.625756719807303,
4.56386006942354));
#11275=CARTESIAN_POINT('Ctrl Pts',(-6.24645857835831,-0.26486761562661,
4.58036302642533));
#11276=CARTESIAN_POINT('Ctrl Pts',(-6.22172441041533,0.176514091733181,
4.59685141347568));
#11277=CARTESIAN_POINT('Ctrl Pts',(-6.43542969978214,0.563067075088938,
4.61332565034683));
#11278=CARTESIAN_POINT('Ctrl Pts',(-6.82170591717644,0.776505131784186,
4.62978623923995));
#11279=CARTESIAN_POINT('Ctrl Pts',(-7.26199738404331,0.75171591878271,4.64623352492646));
#11280=CARTESIAN_POINT('Ctrl Pts',(-7.62128776249611,0.496722562917399,
4.66266823384187));
#11281=CARTESIAN_POINT('Ctrl Pts',(-7.7898227412335,0.0898550976679472,
4.67909025716127));
#11282=CARTESIAN_POINT('Ctrl Pts',(-7.72819305262254,-0.271492440036806,
4.69276624996847));
#11283=CARTESIAN_POINT('Ctrl Pts',(-7.56970306360887,-0.5079089814104,4.70369975196043));
#11284=CARTESIAN_POINT('Ctrl Pts',(-7.35258106881955,-0.69180180336784,
4.71462953902306));
#11285=CARTESIAN_POINT('Ctrl Pts',(-7.00086436408432,-0.793298789487805,
4.7282869636663));
#11286=CARTESIAN_POINT('Ctrl Pts',(-6.5788579709131,-0.671628707119878,
4.74466442804047));
#11287=CARTESIAN_POINT('Ctrl Pts',(-6.28649729752278,-0.344430228222715,
4.76103233022189));
#11288=CARTESIAN_POINT('Ctrl Pts',(-6.21305030592735,0.0879749274087989,
4.77739058654941));
#11289=CARTESIAN_POINT('Ctrl Pts',(-6.38083417398137,0.492926507021418,
4.79373998172835));
#11290=CARTESIAN_POINT('Ctrl Pts',(-6.73816112992995,0.746427111490203,
4.81008089961082));
#11291=CARTESIAN_POINT('Ctrl Pts',(-7.17538345476371,0.770935644450725,
4.82641395115453));
#11292=CARTESIAN_POINT('Ctrl Pts',(-7.55845925877986,0.559185111777055,
4.84273956148575));
#11293=CARTESIAN_POINT('Ctrl Pts',(-7.77008458123184,0.176196391440457,
4.85905846124052));
#11294=CARTESIAN_POINT('Ctrl Pts',(-7.74552463470813,-0.260429333718453,
4.87537080311549));
#11295=CARTESIAN_POINT('Ctrl Pts',(-7.49255708704586,-0.617155518865413,
4.89167805198975));
#11296=CARTESIAN_POINT('Ctrl Pts',(-7.08868802008882,-0.784115034814167,
4.90797883579585));
#11297=CARTESIAN_POINT('Ctrl Pts',(-6.65800791988037,-0.711189244282659,
4.92427325384736));
#11298=CARTESIAN_POINT('Ctrl Pts',(-6.33230245467707,-0.419780727429073,
4.94056584505218));
#11299=CARTESIAN_POINT('Ctrl Pts',(-6.25175641581863,-0.140682475191443,
4.951421508845));
#11300=CARTESIAN_POINT('Ctrl Pts',(-6.2517375291819,-0.000258099276341313,
4.95685288349732));
#11301=CARTESIAN_POINT('Ctrl Pts',(-6.24478965756588,0.00137262626406237,
1.01435596443426));
#11302=CARTESIAN_POINT('Ctrl Pts',(-6.24480872457827,0.143138698890771,
1.01983923355613));
#11303=CARTESIAN_POINT('Ctrl Pts',(-6.32608128465411,0.424978386733189,
1.03079918563777));
#11304=CARTESIAN_POINT('Ctrl Pts',(-6.65521865496514,0.719545141515279,
1.047264334576));
#11305=CARTESIAN_POINT('Ctrl Pts',(-7.09084037841826,0.793351063930433,
1.06374450686311));
#11306=CARTESIAN_POINT('Ctrl Pts',(-7.49970099713228,0.624380947425885,
1.08024415418072));
#11307=CARTESIAN_POINT('Ctrl Pts',(-7.75600750517268,0.263001774579291,
1.096761015804));
#11308=CARTESIAN_POINT('Ctrl Pts',(-7.78094764461577,-0.179705724201667,
1.11329777783683));
#11309=CARTESIAN_POINT('Ctrl Pts',(-7.56624806034485,-0.568359320453272,
1.12985374800478));
#11310=CARTESIAN_POINT('Ctrl Pts',(-7.17722399158054,-0.783435275533458,
1.14642981113991));
#11311=CARTESIAN_POINT('Ctrl Pts',(-6.73292093230953,-0.75857359293873,
1.1630260405376));
#11312=CARTESIAN_POINT('Ctrl Pts',(-6.36935606333102,-0.500772560556008,
1.17964310078603));
#11313=CARTESIAN_POINT('Ctrl Pts',(-6.22723166621629,-0.157314762363655,
1.1935078779172));
#11314=CARTESIAN_POINT('Ctrl Pts',(-6.23575892336378,0.1316270733121,1.20461096131842));
#11315=CARTESIAN_POINT('Ctrl Pts',(-6.32317045688339,0.407351472690643,
1.21572123401303));
#11316=CARTESIAN_POINT('Ctrl Pts',(-6.57129460717402,0.685404517511721,
1.22962200624638));
#11317=CARTESIAN_POINT('Ctrl Pts',(-7.00177871327315,0.809460583789162,
1.24632536995202));
#11318=CARTESIAN_POINT('Ctrl Pts',(-7.43273340799708,0.68539316855628,1.26305104323195));
#11319=CARTESIAN_POINT('Ctrl Pts',(-7.73208724033317,0.350563465410518,
1.27979954233786));
#11320=CARTESIAN_POINT('Ctrl Pts',(-7.80749621963317,-0.0928033737312345,
1.29657108657474));
#11321=CARTESIAN_POINT('Ctrl Pts',(-7.63523348472294,-0.508921058338126,
1.31336601543416));
#11322=CARTESIAN_POINT('Ctrl Pts',(-7.26746462947776,-0.769973596782068,
1.33018460171811));
#11323=CARTESIAN_POINT('Ctrl Pts',(-6.81653894065146,-0.795387340746902,
1.34702713029165));
#11324=CARTESIAN_POINT('Ctrl Pts',(-6.42063877406979,-0.576685808156854,
1.36389386704994));
#11325=CARTESIAN_POINT('Ctrl Pts',(-6.20145878548216,-0.180301041143896,
1.38078506735707));
#11326=CARTESIAN_POINT('Ctrl Pts',(-6.22679890508924,0.272598213463161,
1.39770097937002));
#11327=CARTESIAN_POINT('Ctrl Pts',(-6.48959707258473,0.643145408485334,
1.41464183158308));
#11328=CARTESIAN_POINT('Ctrl Pts',(-6.90988024877083,0.817332105769404,
1.43160785087766));
#11329=CARTESIAN_POINT('Ctrl Pts',(-7.35908439929381,0.741116563166618,
1.44859923602708));
#11330=CARTESIAN_POINT('Ctrl Pts',(-7.69940105999772,0.437104669327555,
1.46561620559972));
#11331=CARTESIAN_POINT('Ctrl Pts',(-7.82599067828337,-0.00196328820679597,
1.48265889161566));
#11332=CARTESIAN_POINT('Ctrl Pts',(-7.69940416409236,-0.441905797127277,
1.4997275794512));
#11333=CARTESIAN_POINT('Ctrl Pts',(-7.41454913261973,-0.69629899338882,
1.51397305883405));
#11334=CARTESIAN_POINT('Ctrl Pts',(-7.13140667031658,-0.786088418557249,
1.52538288124777));
#11335=CARTESIAN_POINT('Ctrl Pts',(-6.83422969008724,-0.794912750226276,
1.53680147993686));
#11336=CARTESIAN_POINT('Ctrl Pts',(-6.49607200192091,-0.654985310754425,
1.55045570442471));
#11337=CARTESIAN_POINT('Ctrl Pts',(-6.2407524690546,-0.317718282519394,
1.56635617473815));
#11338=CARTESIAN_POINT('Ctrl Pts',(-6.18007554423253,0.0841108187200578,
1.58164154787721));
#11339=CARTESIAN_POINT('Ctrl Pts',(-6.31922227546523,0.466683776222355,
1.59694805597311));
#11340=CARTESIAN_POINT('Ctrl Pts',(-6.62482220448134,0.736416004700852,
1.61227569535595));
#11341=CARTESIAN_POINT('Ctrl Pts',(-7.02267006901935,0.827326148404722,
1.62762455399574));
#11342=CARTESIAN_POINT('Ctrl Pts',(-7.41631842058975,0.716646341891919,
1.64299464958104));
#11343=CARTESIAN_POINT('Ctrl Pts',(-7.70898346075156,0.430944328664958,
1.65838604777664));
#11344=CARTESIAN_POINT('Ctrl Pts',(-7.84418225096818,-0.00425490247512673,
1.67551144831122));
#11345=CARTESIAN_POINT('Ctrl Pts',(-7.70153133831721,-0.497784459731678,
1.69437976323737));
#11346=CARTESIAN_POINT('Ctrl Pts',(-7.24499583736429,-0.82620835645191,
1.71500140710803));
#11347=CARTESIAN_POINT('Ctrl Pts',(-6.72987671427024,-0.804517577019736,
1.73393944971573));
#11348=CARTESIAN_POINT('Ctrl Pts',(-6.35763389562258,-0.535974690110675,
1.75118344195896));
#11349=CARTESIAN_POINT('Ctrl Pts',(-6.17818960637836,-0.164043475609255,
1.76672440805754));
#11350=CARTESIAN_POINT('Ctrl Pts',(-6.19876227997895,0.249452063500465,
1.78228670600653));
#11351=CARTESIAN_POINT('Ctrl Pts',(-6.41480376192196,0.603053959900638,
1.79787030241971));
#11352=CARTESIAN_POINT('Ctrl Pts',(-6.77410654704341,0.810584525476164,
1.81347516452805));
#11353=CARTESIAN_POINT('Ctrl Pts',(-7.18964007933331,0.82113897670841,1.82910121659992));
#11354=CARTESIAN_POINT('Ctrl Pts',(-7.49801168006833,0.662761334008476,
1.84214058537142));
#11355=CARTESIAN_POINT('Ctrl Pts',(-7.67730194306007,0.459168604884869,
1.85258264275383));
#11356=CARTESIAN_POINT('Ctrl Pts',(-7.80141394481105,0.217757463993583,
1.86303171269498));
#11357=CARTESIAN_POINT('Ctrl Pts',(-7.83618078765266,-0.128153425658411,
1.87610615924427));
#11358=CARTESIAN_POINT('Ctrl Pts',(-7.67410372643082,-0.513175803930637,
1.89181646036404));
#11359=CARTESIAN_POINT('Ctrl Pts',(-7.34698936491175,-0.774192636346201,
1.90754760602515));
#11360=CARTESIAN_POINT('Ctrl Pts',(-6.96888724945337,-0.840575147748606,
1.92198684917859));
#11361=CARTESIAN_POINT('Ctrl Pts',(-6.63591501935329,-0.751154144255077,
1.93512845763984));
#11362=CARTESIAN_POINT('Ctrl Pts',(-6.38596089432625,-0.566886110545563,
1.94696750823183));
#11363=CARTESIAN_POINT('Ctrl Pts',(-6.2206329095347,-0.303620305915186,
1.95881805136626));
#11364=CARTESIAN_POINT('Ctrl Pts',(-6.16265528038784,0.00213076702521229,
1.97068009034218));
#11365=CARTESIAN_POINT('Ctrl Pts',(-6.22063155782939,0.308074592096969,
1.9825535218887));
#11366=CARTESIAN_POINT('Ctrl Pts',(-6.38639453550796,0.572318399981239,
1.99443833048481));
#11367=CARTESIAN_POINT('Ctrl Pts',(-6.63750082851633,0.757076300713128,
2.00633442846872));
#11368=CARTESIAN_POINT('Ctrl Pts',(-7.03979511845481,0.866354626682583,
2.02221086884604));
#11369=CARTESIAN_POINT('Ctrl Pts',(-7.56452076362568,0.705436392437274,
2.04208449694015));
#11370=CARTESIAN_POINT('Ctrl Pts',(-7.89532063815632,0.132955351120002,
2.06597694663177));
#11371=CARTESIAN_POINT('Ctrl Pts',(-7.74814558033186,-0.512206972690164,
2.08991303508929));
#11372=CARTESIAN_POINT('Ctrl Pts',(-7.20044035770089,-0.885999560658925,
2.11389211328061));
#11373=CARTESIAN_POINT('Ctrl Pts',(-6.54353829697939,-0.787170702788547,
2.13791356135016));
#11374=CARTESIAN_POINT('Ctrl Pts',(-6.12849619905038,-0.267069695319362,
2.1619766919057));
#11375=CARTESIAN_POINT('Ctrl Pts',(-6.17809374798513,0.39764412094938,2.1860807974792));
#11376=CARTESIAN_POINT('Ctrl Pts',(-6.6673876687898,0.851921518939688,2.21022512739177));
#11377=CARTESIAN_POINT('Ctrl Pts',(-7.3361417776358,0.85212632289709,2.23440890190676));
#11378=CARTESIAN_POINT('Ctrl Pts',(-7.82729157862744,0.396676944171653,
2.25863130495804));
#11379=CARTESIAN_POINT('Ctrl Pts',(-7.87761889481913,-0.272298298286383,
2.28289149000321));
#11380=CARTESIAN_POINT('Ctrl Pts',(-7.45885322696456,-0.797717856456593,
2.30718857710582));
#11381=CARTESIAN_POINT('Ctrl Pts',(-6.79351605019779,-0.898187779738267,
2.33152165675313));
#11382=CARTESIAN_POINT('Ctrl Pts',(-6.23665530172092,-0.518743940711026,
2.3558897879953));
#11383=CARTESIAN_POINT('Ctrl Pts',(-6.08633025914367,0.139089740107986,
2.38029200104115));
#11384=CARTESIAN_POINT('Ctrl Pts',(-6.42403744797426,0.724350123935663,
2.40472729859082));
#11385=CARTESIAN_POINT('Ctrl Pts',(-7.07051975136867,0.923937689560396,
2.42919465185401));
#11386=CARTESIAN_POINT('Ctrl Pts',(-7.68095292849436,0.630139560134256,
2.45369301454097));
#11387=CARTESIAN_POINT('Ctrl Pts',(-7.92888975457696,-0.00117722803999169,
2.4782212968774));
#11388=CARTESIAN_POINT('Ctrl Pts',(-7.68096129917293,-0.633397297572642,
2.50277842069243));
#11389=CARTESIAN_POINT('Ctrl Pts',(-7.06847078971012,-0.928413302755619,
2.52736321309282));
#11390=CARTESIAN_POINT('Ctrl Pts',(-6.41822884505462,-0.728138458316165,
2.55197463609316));
#11391=CARTESIAN_POINT('Ctrl Pts',(-6.07724055039059,-0.137772562194659,
2.57661128974893));
#11392=CARTESIAN_POINT('Ctrl Pts',(-6.2041537489263,0.415396542443843,2.59716234881447));
#11393=CARTESIAN_POINT('Ctrl Pts',(-6.5106186599655,0.719851428307833,2.61361411273135));
#11394=CARTESIAN_POINT('Ctrl Pts',(-6.8069155576107,0.849680046560568,2.62595864080187));
#11395=CARTESIAN_POINT('Ctrl Pts',(-7.13082962633578,0.861607082077237,
2.63830854948994));
#11396=CARTESIAN_POINT('Ctrl Pts',(-7.43670743335138,0.754714025872106,
2.650663745239));
#11397=CARTESIAN_POINT('Ctrl Pts',(-7.68242632568281,0.543140860474417,
2.6630240662951));
#11398=CARTESIAN_POINT('Ctrl Pts',(-7.83411705633228,0.256414360912654,
2.67538926259632));
#11399=CARTESIAN_POINT('Ctrl Pts',(-7.87026612947435,-0.0659867172657883,
2.68775937238401));
#11400=CARTESIAN_POINT('Ctrl Pts',(-7.77259819099482,-0.43194811180035,
2.70219621234534));
#11401=CARTESIAN_POINT('Ctrl Pts',(-7.47830389323134,-0.762275469718452,
2.71870351830232));
#11402=CARTESIAN_POINT('Ctrl Pts',(-6.99925195605143,-0.900083285520933,
2.73728406475897));
#11403=CARTESIAN_POINT('Ctrl Pts',(-6.52041326604491,-0.762186110272097,
2.75587330329622));
#11404=CARTESIAN_POINT('Ctrl Pts',(-6.18803904580033,-0.39035034183194,
2.77447098916387));
#11405=CARTESIAN_POINT('Ctrl Pts',(-6.10447020366487,0.10146170411541,2.79307644170198));
#11406=CARTESIAN_POINT('Ctrl Pts',(-6.29542840058373,0.562557359160062,
2.81168919265943));
#11407=CARTESIAN_POINT('Ctrl Pts',(-6.70258147662802,0.851479185427026,
2.83030860229007));
#11408=CARTESIAN_POINT('Ctrl Pts',(-7.20125170285735,0.879494684881194,
2.84893423819587));
#11409=CARTESIAN_POINT('Ctrl Pts',(-7.63843855328058,0.637876372913607,
2.86756526042035));
#11410=CARTESIAN_POINT('Ctrl Pts',(-7.88035809055516,0.200492755901659,
2.88620170890916));
#11411=CARTESIAN_POINT('Ctrl Pts',(-7.85202142204041,-0.29845876402528,
2.90484163379457));
#11412=CARTESIAN_POINT('Ctrl Pts',(-7.56280258302911,-0.706196902313995,
2.92348609265406));
#11413=CARTESIAN_POINT('Ctrl Pts',(-7.10087636837703,-0.897554955048048,
2.94213371595227));
#11414=CARTESIAN_POINT('Ctrl Pts',(-6.60788068228692,-0.813802367473543,
2.96078400814431));
#11415=CARTESIAN_POINT('Ctrl Pts',(-6.23496493305269,-0.480547788919674,
2.97943635760958));
#11416=CARTESIAN_POINT('Ctrl Pts',(-6.09650253414724,7.36349993946475E-5,
2.99809019969138));
#11417=CARTESIAN_POINT('Ctrl Pts',(-6.2349771181594,0.480720839648531,3.01674493477996));
#11418=CARTESIAN_POINT('Ctrl Pts',(-6.60795446695765,0.814029867378355,
3.0353999849881));
#11419=CARTESIAN_POINT('Ctrl Pts',(-7.10108735452254,0.897813287578576,
3.05405475688368));
#11420=CARTESIAN_POINT('Ctrl Pts',(-7.56318811110013,0.706400234832789,
3.07270866751176));
#11421=CARTESIAN_POINT('Ctrl Pts',(-7.85259769038108,0.298505122220334,
3.0913611271422));
#11422=CARTESIAN_POINT('Ctrl Pts',(-7.88062923610225,-0.200789655071514,
3.1100115462463));
#11423=CARTESIAN_POINT('Ctrl Pts',(-7.63875548568654,-0.638405253397185,
3.12865934584202));
#11424=CARTESIAN_POINT('Ctrl Pts',(-7.20120385804123,-0.880216540516199,
3.14730393314355));
#11425=CARTESIAN_POINT('Ctrl Pts',(-6.70216864962299,-0.852175853442006,
3.16594473064668));
#11426=CARTESIAN_POINT('Ctrl Pts',(-6.29463891881066,-0.562996383687711,
3.18458115237288));
#11427=CARTESIAN_POINT('Ctrl Pts',(-6.10347922938325,-0.101444039751134,
3.20321262271211));
#11428=CARTESIAN_POINT('Ctrl Pts',(-6.18715764055134,0.390920015575365,
3.2218385621182));
#11429=CARTESIAN_POINT('Ctrl Pts',(-6.51985614614286,0.763173480128891,
3.24045839411342));
#11430=CARTESIAN_POINT('Ctrl Pts',(-6.99943938334765,0.901311586483643,
3.25907155278571));
#11431=CARTESIAN_POINT('Ctrl Pts',(-7.4788207561827,0.763174459095097,3.27767746322422));
#11432=CARTESIAN_POINT('Ctrl Pts',(-7.81109001430734,0.391318815599289,
3.29627556485821));
#11433=CARTESIAN_POINT('Ctrl Pts',(-7.89455169682821,-0.100097497499467,
3.31486529320673));
#11434=CARTESIAN_POINT('Ctrl Pts',(-7.70386101556373,-0.560374101563154,
3.33344609458917));
#11435=CARTESIAN_POINT('Ctrl Pts',(-7.29772308555257,-0.848499476380384,
3.35201741342008));
#11436=CARTESIAN_POINT('Ctrl Pts',(-6.80081211472958,-0.876366978091514,
3.37057870182124));
#11437=CARTESIAN_POINT('Ctrl Pts',(-6.36548955539379,-0.635727002536597,
3.3891294188677));
#11438=CARTESIAN_POINT('Ctrl Pts',(-6.12506247397863,-0.200625629362112,
3.40766902775647));
#11439=CARTESIAN_POINT('Ctrl Pts',(-6.15296596486626,0.295384481659381,
3.4261969892632));
#11440=CARTESIAN_POINT('Ctrl Pts',(-6.44028359736047,0.700257943509883,
3.44471280120836));
#11441=CARTESIAN_POINT('Ctrl Pts',(-6.89868721845295,0.890065507075794,
3.46321589645446));
#11442=CARTESIAN_POINT('Ctrl Pts',(-7.38738863336506,0.806971596575828,
3.48170588292528));
#11443=CARTESIAN_POINT('Ctrl Pts',(-7.75686478742672,0.476791024583235,
3.50018199886897));
#11444=CARTESIAN_POINT('Ctrl Pts',(-7.87077084655038,0.0804024613658974,
3.51556731136463));
#11445=CARTESIAN_POINT('Ctrl Pts',(-7.82552947727927,-0.23659238310725,
3.52786749975938));
#11446=CARTESIAN_POINT('Ctrl Pts',(-7.69519368038569,-0.5289897821278,3.54016273392284));
#11447=CARTESIAN_POINT('Ctrl Pts',(-7.38837510797035,-0.803387247485029,
3.55552315287051));
#11448=CARTESIAN_POINT('Ctrl Pts',(-6.90118418722867,-0.886299313188514,
3.5739398176403));
#11449=CARTESIAN_POINT('Ctrl Pts',(-6.49650898219159,-0.717941960742899,
3.59029563609768));
#11450=CARTESIAN_POINT('Ctrl Pts',(-6.25206501413344,-0.43331791425204,
3.60459551222303));
#11451=CARTESIAN_POINT('Ctrl Pts',(-6.14579849826547,-0.13015196899678,
3.61684541182134));
#11452=CARTESIAN_POINT('Ctrl Pts',(-6.15795266437509,0.19077242396127,3.62908747996092));
#11453=CARTESIAN_POINT('Ctrl Pts',(-6.28619805958025,0.484932375558522,
3.64132188608379));
#11454=CARTESIAN_POINT('Ctrl Pts',(-6.51307671878171,0.711620993696904,
3.65354829509404));
#11455=CARTESIAN_POINT('Ctrl Pts',(-6.80679521079412,0.839861359046399,
3.66576675059935));
#11456=CARTESIAN_POINT('Ctrl Pts',(-7.12688353097587,0.851781090486876,
3.67797658128607));
#11457=CARTESIAN_POINT('Ctrl Pts',(-7.36183858408272,0.769528777517046,
3.68746696476958));
#11458=CARTESIAN_POINT('Ctrl Pts',(-7.56594880662315,0.634064450549118,
3.69695273716616));
#11459=CARTESIAN_POINT('Ctrl Pts',(-7.75687033874915,0.423412431286683,
3.70778844822587));
#11460=CARTESIAN_POINT('Ctrl Pts',(-7.87355733995844,0.0452323384499969,
3.72267558425976));
#11461=CARTESIAN_POINT('Ctrl Pts',(-7.78447031050978,-0.395461131106034,
3.73957714818353));
#11462=CARTESIAN_POINT('Ctrl Pts',(-7.47096649053771,-0.746487726578873,
3.75713652316082));
#11463=CARTESIAN_POINT('Ctrl Pts',(-7.00154760739981,-0.881615131689879,
3.77535066808487));
#11464=CARTESIAN_POINT('Ctrl Pts',(-6.53288168780712,-0.746479680578851,
3.79354393071519));
#11465=CARTESIAN_POINT('Ctrl Pts',(-6.20824074564234,-0.38313278099757,
3.81171592602832));
#11466=CARTESIAN_POINT('Ctrl Pts',(-6.12683791666095,0.0967518892725567,
3.82986637795763));
#11467=CARTESIAN_POINT('Ctrl Pts',(-6.31289814013408,0.54567365371964,3.84799484839867));
#11468=CARTESIAN_POINT('Ctrl Pts',(-6.70899549333688,0.826886830764423,
3.86610127239849));
#11469=CARTESIAN_POINT('Ctrl Pts',(-7.1391642414818,0.850345684068663,3.88217553454808));
#11470=CARTESIAN_POINT('Ctrl Pts',(-7.4768673421196,0.702589166960476,3.89622519848683));
#11471=CARTESIAN_POINT('Ctrl Pts',(-7.70012720867177,0.479560881685281,
3.90825775646689));
#11472=CARTESIAN_POINT('Ctrl Pts',(-7.82611602300347,0.190439595430187,
3.92027984885091));
#11473=CARTESIAN_POINT('Ctrl Pts',(-7.83798099860797,-0.124443748955779,
3.93229155432904));
#11474=CARTESIAN_POINT('Ctrl Pts',(-7.73390245891118,-0.42146765183984,
3.94429271213602));
#11475=CARTESIAN_POINT('Ctrl Pts',(-7.52878052100635,-0.660108593551094,
3.95628324000648));
#11476=CARTESIAN_POINT('Ctrl Pts',(-7.25098324922026,-0.806353878555257,
3.96826309127496));
#11477=CARTESIAN_POINT('Ctrl Pts',(-6.83480606708229,-0.854597995909426,
3.98422176505027));
#11478=CARTESIAN_POINT('Ctrl Pts',(-6.33885148673084,-0.616373789874939,
4.00414345770479));
#11479=CARTESIAN_POINT('Ctrl Pts',(-6.09743829689286,-0.00172692772890619,
4.02800487858787));
#11480=CARTESIAN_POINT('Ctrl Pts',(-6.33861415409186,0.611112211811564,
4.05182224683903));
#11481=CARTESIAN_POINT('Ctrl Pts',(-6.930890647855,0.896211711923622,4.07559426239331));
#11482=CARTESIAN_POINT('Ctrl Pts',(-7.5578355247161,0.702480238617824,4.09932083585418));
#11483=CARTESIAN_POINT('Ctrl Pts',(-7.88507859972884,0.135449505681517,
4.12300136072554));
#11484=CARTESIAN_POINT('Ctrl Pts',(-7.73933983592004,-0.502118403477305,
4.14663556803947));
#11485=CARTESIAN_POINT('Ctrl Pts',(-7.26039367113424,-0.827655820518871,
4.16760211727223));
#11486=CARTESIAN_POINT('Ctrl Pts',(-6.77288173277215,-0.813828340996825,
4.18591758737132));
#11487=CARTESIAN_POINT('Ctrl Pts',(-6.41210932711652,-0.605956030043776,
4.20159558574628));
#11488=CARTESIAN_POINT('Ctrl Pts',(-6.19501402257771,-0.250376696431912,
4.21725247157529));
#11489=CARTESIAN_POINT('Ctrl Pts',(-6.17417056259732,0.164760155164131,
4.23288813280655));
#11490=CARTESIAN_POINT('Ctrl Pts',(-6.3545942969234,0.538855542040888,4.24850255309216));
#11491=CARTESIAN_POINT('Ctrl Pts',(-6.66328617817794,0.760507888724256,
4.26279661491745));
#11492=CARTESIAN_POINT('Ctrl Pts',(-6.9978784626736,0.823569792509618,4.27577535769565));
#11493=CARTESIAN_POINT('Ctrl Pts',(-7.29866400314611,0.766751391781709,
4.28744432659339));
#11494=CARTESIAN_POINT('Ctrl Pts',(-7.55744540147431,0.603995266851033,
4.29910128219956));
#11495=CARTESIAN_POINT('Ctrl Pts',(-7.73905541731227,0.358135252089175,
4.31074622431009));
#11496=CARTESIAN_POINT('Ctrl Pts',(-7.81749152608428,0.0636809190910327,
4.3223791871992));
#11497=CARTESIAN_POINT('Ctrl Pts',(-7.77317917381171,-0.341116140474648,
4.33787368203927));
#11498=CARTESIAN_POINT('Ctrl Pts',(-7.50721032388302,-0.674391183617128,
4.35334442702289));
#11499=CARTESIAN_POINT('Ctrl Pts',(-7.12360277329797,-0.807159429383535,
4.36879085079072));
#11500=CARTESIAN_POINT('Ctrl Pts',(-6.82064966915069,-0.79622001697244,
4.38036369654546));
#11501=CARTESIAN_POINT('Ctrl Pts',(-6.54258356263728,-0.674699950250188,
4.39192452633223));
#11502=CARTESIAN_POINT('Ctrl Pts',(-6.32838183258931,-0.460587210838161,
4.40347334046582));
#11503=CARTESIAN_POINT('Ctrl Pts',(-6.20745638360056,-0.183141123111028,
4.4150101887781));
#11504=CARTESIAN_POINT('Ctrl Pts',(-6.19607090850112,0.118985454375757,
4.42653502983482));
#11505=CARTESIAN_POINT('Ctrl Pts',(-6.29598849817137,0.40391719529154,4.43804794900205));
#11506=CARTESIAN_POINT('Ctrl Pts',(-6.52539085352358,0.670952624756736,
4.45146570163604));
#11507=CARTESIAN_POINT('Ctrl Pts',(-6.90442160364007,0.828498869433625,
4.46678049304922));
#11508=CARTESIAN_POINT('Ctrl Pts',(-7.35937715782801,0.75087237148055,4.48398292034035));
#11509=CARTESIAN_POINT('Ctrl Pts',(-7.70263994562715,0.444003510586905,
4.50115870290066));
#11510=CARTESIAN_POINT('Ctrl Pts',(-7.82989303341533,0.00204106946231624,
4.51830796948457));
#11511=CARTESIAN_POINT('Ctrl Pts',(-7.70267552148953,-0.43911345287367,
4.53543083756206));
#11512=CARTESIAN_POINT('Ctrl Pts',(-7.36078794810659,-0.74453315607766,
4.55252744875789));
#11513=CARTESIAN_POINT('Ctrl Pts',(-6.90949624334495,-0.821109089414126,
4.56959794960374));
#11514=CARTESIAN_POINT('Ctrl Pts',(-6.48728069604972,-0.646119024648585,
4.58664250216479));
#11515=CARTESIAN_POINT('Ctrl Pts',(-6.22328014245951,-0.273879047789936,
4.60366128068545));
#11516=CARTESIAN_POINT('Ctrl Pts',(-6.19782444473162,0.181078373118608,
4.62065446856178));
#11517=CARTESIAN_POINT('Ctrl Pts',(-6.41799641702055,0.5792458930126,4.63762226650895));
#11518=CARTESIAN_POINT('Ctrl Pts',(-6.81565826960756,0.798929031456019,
4.6545648765693));
#11519=CARTESIAN_POINT('Ctrl Pts',(-7.26859902401305,0.773385786288969,
4.67148253456703));
#11520=CARTESIAN_POINT('Ctrl Pts',(-7.63793616170917,0.511211936303308,
4.68837544184199));
#11521=CARTESIAN_POINT('Ctrl Pts',(-7.81103129278376,0.0932135444940163,
4.7052439075552));
#11522=CARTESIAN_POINT('Ctrl Pts',(-7.74772659633056,-0.277723366438459,
4.71928068135095));
#11523=CARTESIAN_POINT('Ctrl Pts',(-7.58510165644112,-0.520294036256702,
4.73049830024372));
#11524=CARTESIAN_POINT('Ctrl Pts',(-7.36239850996586,-0.708904500801799,
4.74170798257738));
#11525=CARTESIAN_POINT('Ctrl Pts',(-7.00186095481488,-0.812908884827261,
4.75570503351309));
#11526=CARTESIAN_POINT('Ctrl Pts',(-6.56961433191529,-0.688237747232737,
4.77247823631829));
#11527=CARTESIAN_POINT('Ctrl Pts',(-6.27042017705918,-0.353314214709758,
4.78922830449849));
#11528=CARTESIAN_POINT('Ctrl Pts',(-6.19535597538779,0.0889191605106485,
4.80595562242244));
#11529=CARTESIAN_POINT('Ctrl Pts',(-6.36686335581866,0.502719028652008,
4.8226604694237));
#11530=CARTESIAN_POINT('Ctrl Pts',(-6.73175256486973,0.761520072268675,
4.83934320448615));
#11531=CARTESIAN_POINT('Ctrl Pts',(-7.17782997977493,0.786473326771477,
4.85600412593016));
#11532=CARTESIAN_POINT('Ctrl Pts',(-7.5683126081094,0.57057171907611,4.87264365440957));
#11533=CARTESIAN_POINT('Ctrl Pts',(-7.78382263552961,0.180461387737065,
4.88926197808321));
#11534=CARTESIAN_POINT('Ctrl Pts',(-7.75878282229075,-0.263872752181399,
4.90585981848288));
#11535=CARTESIAN_POINT('Ctrl Pts',(-7.50154978164387,-0.626551986690765,
4.92243671953082));
#11536=CARTESIAN_POINT('Ctrl Pts',(-7.09124424921979,-0.796114951309141,
4.93899483030102));
#11537=CARTESIAN_POINT('Ctrl Pts',(-6.65411810003208,-0.722048191241108,
4.95553216226915));
#11538=CARTESIAN_POINT('Ctrl Pts',(-6.32387059158365,-0.426484570176635,
4.97205308357914));
#11539=CARTESIAN_POINT('Ctrl Pts',(-6.24232917383988,-0.143709849746694,
4.98304959780136));
#11540=CARTESIAN_POINT('Ctrl Pts',(-6.24231004509627,-0.00148538057916514,
4.98855059698146));
#11541=CARTESIAN_POINT('Ctrl Pts',(-6.25574144158882,-0.000498857481043991,
1.06270377973105));
#11542=CARTESIAN_POINT('Ctrl Pts',(-6.25576022828242,0.139183003238407,
1.06810643510251));
#11543=CARTESIAN_POINT('Ctrl Pts',(-6.33586682667619,0.416721998384859,
1.07890094002148));
#11544=CARTESIAN_POINT('Ctrl Pts',(-6.65959485848297,0.706318708188977,
1.09509298618406));
#11545=CARTESIAN_POINT('Ctrl Pts',(-7.08739810828336,0.778721847560845,
1.11127784875485));
#11546=CARTESIAN_POINT('Ctrl Pts',(-7.48832794984565,0.612939978136046,
1.1274597570632));
#11547=CARTESIAN_POINT('Ctrl Pts',(-7.73928794456948,0.258977919487233,
1.14363817134105));
#11548=CARTESIAN_POINT('Ctrl Pts',(-7.76360338401286,-0.174005578196651,
1.15981328783718));
#11549=CARTESIAN_POINT('Ctrl Pts',(-7.55383634477513,-0.553573253430915,
1.17598591488793));
#11550=CARTESIAN_POINT('Ctrl Pts',(-7.17433261104523,-0.76329584980855,
1.19215651921613));
#11551=CARTESIAN_POINT('Ctrl Pts',(-6.74151458194365,-0.738996757692014,
1.20832585703833));
#11552=CARTESIAN_POINT('Ctrl Pts',(-6.38784581103617,-0.488116990817084,
1.22449424575166));
#11553=CARTESIAN_POINT('Ctrl Pts',(-6.24980489864987,-0.15436255814959,
1.23796812666697));
#11554=CARTESIAN_POINT('Ctrl Pts',(-6.25809489187119,0.126118231152519,
1.24874671827879));
#11555=CARTESIAN_POINT('Ctrl Pts',(-6.34290773639547,0.393603166796141,
1.25952554349459));
#11556=CARTESIAN_POINT('Ctrl Pts',(-6.58345162450279,0.663066705711368,
1.27300057006987));
#11557=CARTESIAN_POINT('Ctrl Pts',(-7.00020483358905,0.783086765045414,
1.28917173167979));
#11558=CARTESIAN_POINT('Ctrl Pts',(-7.41687065522309,0.663059338011621,
1.30534521235595));
#11559=CARTESIAN_POINT('Ctrl Pts',(-7.70591544232305,0.339653901481795,
1.3215213522553));
#11560=CARTESIAN_POINT('Ctrl Pts',(-7.77858712938061,-0.0880332025193281,
1.33770084993892));
#11561=CARTESIAN_POINT('Ctrl Pts',(-7.61254839496213,-0.488936729999324,
1.35388424102803));
#11562=CARTESIAN_POINT('Ctrl Pts',(-7.25856334262776,-0.740122115944731,
1.37007213360199));
#11563=CARTESIAN_POINT('Ctrl Pts',(-6.82506267309524,-0.764487181544599,
1.38626509399126));
#11564=CARTESIAN_POINT('Ctrl Pts',(-6.44490903164376,-0.554409724240902,
1.40246370734102));
#11565=CARTESIAN_POINT('Ctrl Pts',(-6.23470889983783,-0.174132948159932,
1.41866854181864));
#11566=CARTESIAN_POINT('Ctrl Pts',(-6.25905438180472,0.259870837709405,
1.43488017508944));
#11567=CARTESIAN_POINT('Ctrl Pts',(-6.51068392324855,0.614564502512315,
1.45109917288617));
#11568=CARTESIAN_POINT('Ctrl Pts',(-6.91264883964463,0.78109446323033,1.46732609435233));
#11569=CARTESIAN_POINT('Ctrl Pts',(-7.34182339671781,0.708217790535654,
1.48356152351232));
#11570=CARTESIAN_POINT('Ctrl Pts',(-7.66662800022932,0.417986725042806,
1.49980597216501));
#11571=CARTESIAN_POINT('Ctrl Pts',(-7.7872969698189,-0.000747736846312889,
1.51606009973265));
#11572=CARTESIAN_POINT('Ctrl Pts',(-7.6666342868507,-0.419909780883938,
1.53232423514785));
#11573=CARTESIAN_POINT('Ctrl Pts',(-7.39543041252767,-0.662055716649145,
1.54588691377005));
#11574=CARTESIAN_POINT('Ctrl Pts',(-7.12606123934068,-0.747468998803105,
1.55674207242413));
#11575=CARTESIAN_POINT('Ctrl Pts',(-6.84345620821393,-0.755852189904183,
1.56760104700489));
#11576=CARTESIAN_POINT('Ctrl Pts',(-6.5220837749257,-0.622828513848678,
1.58057931637516));
#11577=CARTESIAN_POINT('Ctrl Pts',(-6.27964104193747,-0.302511596729687,
1.59568049942823));
#11578=CARTESIAN_POINT('Ctrl Pts',(-6.2220864354709,0.0788440259113018,
1.61018790303456));
#11579=CARTESIAN_POINT('Ctrl Pts',(-6.35408418226561,0.441670066477265,
1.62470565559779));
#11580=CARTESIAN_POINT('Ctrl Pts',(-6.64375339876684,0.697301801776668,
1.63923425150086));
#11581=CARTESIAN_POINT('Ctrl Pts',(-7.0206119357728,0.783386360219316,1.65377397435476));
#11582=CARTESIAN_POINT('Ctrl Pts',(-7.39325720437512,0.678581967567608,
1.6683252500628));
#11583=CARTESIAN_POINT('Ctrl Pts',(-7.67013870264448,0.408254260386592,
1.68288834541239));
#11584=CARTESIAN_POINT('Ctrl Pts',(-7.79795365163416,-0.0032820587900806,
1.6990827439662));
#11585=CARTESIAN_POINT('Ctrl Pts',(-7.66309442919013,-0.469667500024928,
1.71691460045667));
#11586=CARTESIAN_POINT('Ctrl Pts',(-7.23190668680682,-0.779785048350367,
1.73639051607248));
#11587=CARTESIAN_POINT('Ctrl Pts',(-6.74573184654296,-0.759267380311345,
1.75426513540613));
#11588=CARTESIAN_POINT('Ctrl Pts',(-6.39459107302207,-0.505920169111814,
1.77053310370253));
#11589=CARTESIAN_POINT('Ctrl Pts',(-6.2253973160446,-0.155195481687715,
1.7851883329396));
#11590=CARTESIAN_POINT('Ctrl Pts',(-6.24480623004818,0.234563730110018,
1.79985798765964));
#11591=CARTESIAN_POINT('Ctrl Pts',(-6.44838629115469,0.567738725777836,
1.81454239612435));
#11592=CARTESIAN_POINT('Ctrl Pts',(-6.78683423413161,0.763206916772546,
1.82924177771278));
#11593=CARTESIAN_POINT('Ctrl Pts',(-7.17811932257024,0.773131221068672,
1.84395664824561));
#11594=CARTESIAN_POINT('Ctrl Pts',(-7.46840416020655,0.6240316513085,1.8562317924873));
#11595=CARTESIAN_POINT('Ctrl Pts',(-7.63714510399363,0.432414888572534,
1.86605972191242));
#11596=CARTESIAN_POINT('Ctrl Pts',(-7.75393931700189,0.205233365517019,
1.8758930057902));
#11597=CARTESIAN_POINT('Ctrl Pts',(-7.78664215748584,-0.120233197607642,
1.88819523160421));
#11598=CARTESIAN_POINT('Ctrl Pts',(-7.63417045939035,-0.482409153902618,
1.90297364848866));
#11599=CARTESIAN_POINT('Ctrl Pts',(-7.32651359382278,-0.72789070482646,
1.91776950585886));
#11600=CARTESIAN_POINT('Ctrl Pts',(-6.97097117673883,-0.790305576233221,
1.93134746236838));
#11601=CARTESIAN_POINT('Ctrl Pts',(-6.65790957425775,-0.706229485674086,
1.94370343248341));
#11602=CARTESIAN_POINT('Ctrl Pts',(-6.42292495799198,-0.532993864392855,
1.95483369581103));
#11603=CARTESIAN_POINT('Ctrl Pts',(-6.26751159004392,-0.285514108223224,
1.96597379393668));
#11604=CARTESIAN_POINT('Ctrl Pts',(-6.21301625364804,0.00188292046488118,
1.97712387179597));
#11605=CARTESIAN_POINT('Ctrl Pts',(-6.2675090658162,0.289443762118776,1.98828402919144));
#11606=CARTESIAN_POINT('Ctrl Pts',(-6.42330583078288,0.537798456401413,
1.99945431517307));
#11607=CARTESIAN_POINT('Ctrl Pts',(-6.65930551885432,0.7114420938548,2.01063488878302));
#11608=CARTESIAN_POINT('Ctrl Pts',(-7.03739094524968,0.814143836989083,
2.02555601312736));
#11609=CARTESIAN_POINT('Ctrl Pts',(-7.53053768011085,0.662913683709486,
2.04423381193589));
#11610=CARTESIAN_POINT('Ctrl Pts',(-7.84144903768382,0.124870379518979,
2.06668933863783));
#11611=CARTESIAN_POINT('Ctrl Pts',(-7.70312872983905,-0.481547002699999,
2.0891879441913));
#11612=CARTESIAN_POINT('Ctrl Pts',(-7.1882562937634,-0.832958294320995,
2.11173012604567));
#11613=CARTESIAN_POINT('Ctrl Pts',(-6.57059338007734,-0.740060748597092,
2.13431650032462));
#11614=CARTESIAN_POINT('Ctrl Pts',(-6.1802232556478,-0.250930801799442,
2.15694757743791));
#11615=CARTESIAN_POINT('Ctrl Pts',(-6.22684370912928,0.374415923588821,
2.17962385701603));
#11616=CARTESIAN_POINT('Ctrl Pts',(-6.68728605866362,0.801968733566327,
2.20234578920383));
#11617=CARTESIAN_POINT('Ctrl Pts',(-7.31689820140758,0.802213040629406,
2.22511378940577));
#11618=CARTESIAN_POINT('Ctrl Pts',(-7.77954577036186,0.373272342681926,
2.24792823286914));
#11619=CARTESIAN_POINT('Ctrl Pts',(-7.82703482894681,-0.257133770025224,
2.27078945587098));
#11620=CARTESIAN_POINT('Ctrl Pts',(-7.43225046320483,-0.752574828411877,
2.29369775546632));
#11621=CARTESIAN_POINT('Ctrl Pts',(-6.80457236171091,-0.847433409521687,
2.31665338874161));
#11622=CARTESIAN_POINT('Ctrl Pts',(-6.27884387479177,-0.489300063191618,
2.33965657329448));
#11623=CARTESIAN_POINT('Ctrl Pts',(-6.13675540828559,0.132104889847011,
2.36270748645569));
#11624=CARTESIAN_POINT('Ctrl Pts',(-6.45592275124396,0.685417394331864,
2.38580626524834));
#11625=CARTESIAN_POINT('Ctrl Pts',(-7.06750462557763,0.874331252516317,
2.40895300717511));
#11626=CARTESIAN_POINT('Ctrl Pts',(-7.64552182519084,0.596247683724882,
2.43214776683914));
#11627=CARTESIAN_POINT('Ctrl Pts',(-7.88057376599971,-0.00196814628072304,
2.45539056393457));
#11628=CARTESIAN_POINT('Ctrl Pts',(-7.64552409477716,-0.601654948176037,
2.47868136373957));
#11629=CARTESIAN_POINT('Ctrl Pts',(-7.06410018348824,-0.881837376955094,
2.50202012163737));
#11630=CARTESIAN_POINT('Ctrl Pts',(-6.44615034947898,-0.691637521520468,
2.52540667870236));
#11631=CARTESIAN_POINT('Ctrl Pts',(-6.12167515050772,-0.130120742172608,
2.54884100103956));
#11632=CARTESIAN_POINT('Ctrl Pts',(-6.24242004156193,0.396652017996355,
2.56840901450238));
#11633=CARTESIAN_POINT('Ctrl Pts',(-6.53447535363075,0.686823681480564,
2.58408734767232));
#11634=CARTESIAN_POINT('Ctrl Pts',(-6.81699805059676,0.810635681023223,
2.59585781985285));
#11635=CARTESIAN_POINT('Ctrl Pts',(-7.12603611624708,0.822030492458687,
2.60764008421422));
#11636=CARTESIAN_POINT('Ctrl Pts',(-7.41803788514657,0.72000683301485,2.61943404873999));
#11637=CARTESIAN_POINT('Ctrl Pts',(-7.65274995755222,0.517929884868489,
2.63123970145475));
#11638=CARTESIAN_POINT('Ctrl Pts',(-7.79774172107598,0.243906477114829,
2.64305702599696));
#11639=CARTESIAN_POINT('Ctrl Pts',(-7.83232527997599,-0.0644032051053991,
2.65488589026192));
#11640=CARTESIAN_POINT('Ctrl Pts',(-7.73889023355586,-0.414589190311789,
2.66869990431192));
#11641=CARTESIAN_POINT('Ctrl Pts',(-7.45711558261939,-0.730943004383703,
2.68450617152468));
#11642=CARTESIAN_POINT('Ctrl Pts',(-6.99796978668839,-0.863090579444672,
2.70231373581129));
#11643=CARTESIAN_POINT('Ctrl Pts',(-6.53855217084151,-0.730852022510803,
2.72014697009195));
#11644=CARTESIAN_POINT('Ctrl Pts',(-6.21931412255978,-0.373809109467704,
2.73800549127301));
#11645=CARTESIAN_POINT('Ctrl Pts',(-6.13891465776656,0.0989486782214521,
2.7558891571914));
#11646=CARTESIAN_POINT('Ctrl Pts',(-6.32259891652746,0.542660491028362,
2.77379768621757));
#11647=CARTESIAN_POINT('Ctrl Pts',(-6.71473487923161,0.821012435181475,
2.79173089130173));
#11648=CARTESIAN_POINT('Ctrl Pts',(-7.19555373615558,0.848098151534184,
2.80968842316349));
#11649=CARTESIAN_POINT('Ctrl Pts',(-7.61756823154174,0.614945844011524,
2.82767022347362));
#11650=CARTESIAN_POINT('Ctrl Pts',(-7.85138514701445,0.192369550326599,
2.84567556880744));
#11651=CARTESIAN_POINT('Ctrl Pts',(-7.82404608394165,-0.290269192588259,
2.86370517231971));
#11652=CARTESIAN_POINT('Ctrl Pts',(-7.54405162406482,-0.685136423624603,
2.88175754722335));
#11653=CARTESIAN_POINT('Ctrl Pts',(-7.09629257868619,-0.870707936190149,
2.89983297266089));
#11654=CARTESIAN_POINT('Ctrl Pts',(-6.61784180407662,-0.789503998643947,
2.91793106339489));
#11655=CARTESIAN_POINT('Ctrl Pts',(-6.25547880694769,-0.465783876765169,
2.9360515100578));
#11656=CARTESIAN_POINT('Ctrl Pts',(-6.12072563265172,0.00167905711825161,
2.95419397011278));
#11657=CARTESIAN_POINT('Ctrl Pts',(-6.25549336745657,0.46974689465823,2.97235809483517));
#11658=CARTESIAN_POINT('Ctrl Pts',(-6.61905883922182,0.794752880995018,
2.9905435289329));
#11659=CARTESIAN_POINT('Ctrl Pts',(-7.10036600226087,0.876609499720008,
3.0087499032196));
#11660=CARTESIAN_POINT('Ctrl Pts',(-7.55195993204527,0.689637344969144,
3.0269768429918));
#11661=CARTESIAN_POINT('Ctrl Pts',(-7.83517221510059,0.29061953446048,3.04522396103687));
#11662=CARTESIAN_POINT('Ctrl Pts',(-7.86271284952522,-0.198445949703901,
3.06349085934156));
#11663=CARTESIAN_POINT('Ctrl Pts',(-7.6255807553781,-0.627655924321167,
3.08177713801619));
#11664=CARTESIAN_POINT('Ctrl Pts',(-7.19599570183822,-0.865160948375789,
3.100082377186));
#11665=CARTESIAN_POINT('Ctrl Pts',(-6.70539880249602,-0.837679482344607,
3.11840615795295));
#11666=CARTESIAN_POINT('Ctrl Pts',(-6.30422426083902,-0.553114363892535,
3.13674804536529));
#11667=CARTESIAN_POINT('Ctrl Pts',(-6.11575799788189,-0.0982897902643771,
3.15510760179694));
#11668=CARTESIAN_POINT('Ctrl Pts',(-6.19823939872231,0.387546459541662,
3.17348437694896));
#11669=CARTESIAN_POINT('Ctrl Pts',(-6.52685982154688,0.755367181396514,
3.19187791210836));
#11670=CARTESIAN_POINT('Ctrl Pts',(-7.00122376758996,0.892092600222727,
3.21028774728281));
#11671=CARTESIAN_POINT('Ctrl Pts',(-7.47602897177808,0.755365132384686,
3.22871340448373));
#11672=CARTESIAN_POINT('Ctrl Pts',(-7.80558752389931,0.386674816692687,
3.24715440718115));
#11673=CARTESIAN_POINT('Ctrl Pts',(-7.8885426204605,-0.101233380981048,
3.26561026530892));
#11674=CARTESIAN_POINT('Ctrl Pts',(-7.69905050675687,-0.558847314582516,
3.28408048670801));
#11675=CARTESIAN_POINT('Ctrl Pts',(-7.29483346934859,-0.845718266442943,
3.3025645681768));
#11676=CARTESIAN_POINT('Ctrl Pts',(-6.79959008958347,-0.873580860447485,
3.32106199909265));
#11677=CARTESIAN_POINT('Ctrl Pts',(-6.36513240365607,-0.633520245208162,
3.33957227042389));
#11678=CARTESIAN_POINT('Ctrl Pts',(-6.12482522958441,-0.198819481209487,
3.35809485071837));
#11679=CARTESIAN_POINT('Ctrl Pts',(-6.15265228854888,0.297415232772545,
3.37662922508223));
#11680=CARTESIAN_POINT('Ctrl Pts',(-6.44038811710877,0.703032318644318,
3.39517483032209));
#11681=CARTESIAN_POINT('Ctrl Pts',(-6.90012184892277,0.893486914765094,
3.41373118314646));
#11682=CARTESIAN_POINT('Ctrl Pts',(-7.39091111614474,0.81012884982552,3.43229760104649));
#11683=CARTESIAN_POINT('Ctrl Pts',(-7.76248245627454,0.478194158159316,
3.45087381180285));
#11684=CARTESIAN_POINT('Ctrl Pts',(-7.87722924504625,0.0791422613117201,
3.4663611170865));
#11685=CARTESIAN_POINT('Ctrl Pts',(-7.83165133922849,-0.240314783834962,
3.47875598768671));
#11686=CARTESIAN_POINT('Ctrl Pts',(-7.70023907701898,-0.535167149935524,
3.49115356884793));
#11687=CARTESIAN_POINT('Ctrl Pts',(-7.39062087111684,-0.812170012694234,
3.50665454205289));
#11688=CARTESIAN_POINT('Ctrl Pts',(-6.89830560717456,-0.896052546468553,
3.52526326778163));
#11689=CARTESIAN_POINT('Ctrl Pts',(-6.48880985910723,-0.725774650674278,
3.54181063235856));
#11690=CARTESIAN_POINT('Ctrl Pts',(-6.24118965329123,-0.437496870629759,
3.55629441767643));
#11691=CARTESIAN_POINT('Ctrl Pts',(-6.13343726805911,-0.130184025345005,
3.5687112475538));
#11692=CARTESIAN_POINT('Ctrl Pts',(-6.14574491655201,0.195411889709324,
3.58113072282879));
#11693=CARTESIAN_POINT('Ctrl Pts',(-6.27593308314913,0.494106501635381,
3.59355230196842));
#11694=CARTESIAN_POINT('Ctrl Pts',(-6.50647484898252,0.72448430278658,3.60597607343073));
#11695=CARTESIAN_POINT('Ctrl Pts',(-6.80518220959668,0.854933539558384,
3.61840163759416));
#11696=CARTESIAN_POINT('Ctrl Pts',(-7.13099645393491,0.867086944731104,
3.6308294909089));
#11697=CARTESIAN_POINT('Ctrl Pts',(-7.37034629814982,0.78331581805002,3.64049644697034));
#11698=CARTESIAN_POINT('Ctrl Pts',(-7.57838611791206,0.645242841704105,
3.65016442339402));
#11699=CARTESIAN_POINT('Ctrl Pts',(-7.77310581402586,0.430433141736348,
3.6612145176939));
#11700=CARTESIAN_POINT('Ctrl Pts',(-7.89226187454386,0.0444204254824345,
3.67640971635602));
#11701=CARTESIAN_POINT('Ctrl Pts',(-7.80129086431032,-0.405895837677021,
3.69367799765519));
#11702=CARTESIAN_POINT('Ctrl Pts',(-7.48064329455355,-0.76503136866683,
3.71163847341778));
#11703=CARTESIAN_POINT('Ctrl Pts',(-6.99989620560288,-0.903501260319285,
3.73029091807058));
#11704=CARTESIAN_POINT('Ctrl Pts',(-6.51931206875194,-0.765010981613905,
3.74894385066014));
#11705=CARTESIAN_POINT('Ctrl Pts',(-6.18598457115065,-0.392062541037647,
3.7675966949923));
#11706=CARTESIAN_POINT('Ctrl Pts',(-6.10224048559192,0.101126455191569,
3.78624875991382));
#11707=CARTESIAN_POINT('Ctrl Pts',(-6.29360664053959,0.563061899641102,
3.80489957562934));
#11708=CARTESIAN_POINT('Ctrl Pts',(-6.70156274884057,0.852798275855841,
3.82354818129352));
#11709=CARTESIAN_POINT('Ctrl Pts',(-7.14516419629844,0.877060146522431,
3.84012284280759));
#11710=CARTESIAN_POINT('Ctrl Pts',(-7.49375117715357,0.724569432080486,
3.85462433846513));
#11711=CARTESIAN_POINT('Ctrl Pts',(-7.72438066713674,0.494215522957976,
3.86705226830291));
#11712=CARTESIAN_POINT('Ctrl Pts',(-7.8546314996621,0.195364139195026,3.87947864210889));
#11713=CARTESIAN_POINT('Ctrl Pts',(-7.86693096726382,-0.130355958792914,
3.89190302709772));
#11714=CARTESIAN_POINT('Ctrl Pts',(-7.75920990140556,-0.437827963480458,
3.90432538766937));
#11715=CARTESIAN_POINT('Ctrl Pts',(-7.54674669970804,-0.685049391800177,
3.91674551833732));
#11716=CARTESIAN_POINT('Ctrl Pts',(-7.2587832470136,-0.836663148820833,
3.92916323122733));
#11717=CARTESIAN_POINT('Ctrl Pts',(-6.82707910403541,-0.886741311123473,
3.94571687930683));
#11718=CARTESIAN_POINT('Ctrl Pts',(-6.31203054929912,-0.639493595762034,
3.966401355575));
#11719=CARTESIAN_POINT('Ctrl Pts',(-6.06084279300897,-0.000449608345310296,
3.99121135126554));
#11720=CARTESIAN_POINT('Ctrl Pts',(-6.31179693592123,0.637682779121499,
4.01600691862606));
#11721=CARTESIAN_POINT('Ctrl Pts',(-6.92918191266279,0.935049780651178,
4.04078798038478));
#11722=CARTESIAN_POINT('Ctrl Pts',(-7.58365238518735,0.732979239453076,
4.06555261138874));
#11723=CARTESIAN_POINT('Ctrl Pts',(-7.9257900806735,0.140447811970743,4.09029979894177));
#11724=CARTESIAN_POINT('Ctrl Pts',(-7.77344406870196,-0.526712992467699,
4.11502804101992));
#11725=CARTESIAN_POINT('Ctrl Pts',(-7.27177779124963,-0.867844577177589,
4.13699100638644));
#11726=CARTESIAN_POINT('Ctrl Pts',(-6.76058665329715,-0.853396344821666,
4.15619430386727));
#11727=CARTESIAN_POINT('Ctrl Pts',(-6.38200074112008,-0.635302741652714,
4.1726443652993));
#11728=CARTESIAN_POINT('Ctrl Pts',(-6.15400141844129,-0.261934603150095,
4.18908432068376));
#11729=CARTESIAN_POINT('Ctrl Pts',(-6.13205747172757,0.174301185046141,
4.20551384069495));
#11730=CARTESIAN_POINT('Ctrl Pts',(-6.32175295930821,0.567698027428144,
4.22193258418429));
#11731=CARTESIAN_POINT('Ctrl Pts',(-6.64654841184092,0.800957389537971,
4.23697195571088));
#11732=CARTESIAN_POINT('Ctrl Pts',(-6.99882766587418,0.867367090001126,
4.25063646985522));
#11733=CARTESIAN_POINT('Ctrl Pts',(-7.31566615380246,0.807532578123425,
4.26292758526584));
#11734=CARTESIAN_POINT('Ctrl Pts',(-7.58839195679831,0.636020296619523,
4.27521192630173));
#11735=CARTESIAN_POINT('Ctrl Pts',(-7.77988431286369,0.37680928883101,4.28748926184605));
#11736=CARTESIAN_POINT('Ctrl Pts',(-7.8626299224257,0.0662152386377366,
4.29975939205125));
#11737=CARTESIAN_POINT('Ctrl Pts',(-7.81589040587151,-0.360959854603563,
4.31611012161726));
#11738=CARTESIAN_POINT('Ctrl Pts',(-7.53509133921148,-0.71291947800451,
4.33244512578823));
#11739=CARTESIAN_POINT('Ctrl Pts',(-7.12976760986697,-0.85322217354558,
4.34876566200336));
#11740=CARTESIAN_POINT('Ctrl Pts',(-6.80953724060416,-0.841669304187541,
4.36099807640831));
#11741=CARTESIAN_POINT('Ctrl Pts',(-6.51549418290265,-0.713177572198111,
4.3732226080825));
#11742=CARTESIAN_POINT('Ctrl Pts',(-6.2888947681933,-0.486688725403999,
4.38543907223306));
#11743=CARTESIAN_POINT('Ctrl Pts',(-6.160920555938,-0.193090427094334,4.39764730462965));
#11744=CARTESIAN_POINT('Ctrl Pts',(-6.14885699254258,0.126741694206413,
4.40984729976258));
#11745=CARTESIAN_POINT('Ctrl Pts',(-6.25465979225549,0.428478434738072,
4.42203873484718));
#11746=CARTESIAN_POINT('Ctrl Pts',(-6.49766240970981,0.711363326767944,
4.43625235165378));
#11747=CARTESIAN_POINT('Ctrl Pts',(-6.89932724358013,0.878345874150377,
4.45248156448681));
#11748=CARTESIAN_POINT('Ctrl Pts',(-7.38168762889607,0.796072531346823,
4.47071928201173));
#11749=CARTESIAN_POINT('Ctrl Pts',(-7.74579952770647,0.470600467593104,
4.48893682127011));
#11750=CARTESIAN_POINT('Ctrl Pts',(-7.88085359657661,0.00163419859513053,
4.50713360807125));
#11751=CARTESIAN_POINT('Ctrl Pts',(-7.74583271530823,-0.466665339744885,
4.52530933877659));
#11752=CARTESIAN_POINT('Ctrl Pts',(-7.38280065073972,-0.791003440257137,
4.54346360414915));
#11753=CARTESIAN_POINT('Ctrl Pts',(-6.90342748857269,-0.872364778276333,
4.56159606648756));
#11754=CARTESIAN_POINT('Ctrl Pts',(-6.45479686015966,-0.686446622036828,
4.57970637146554));
#11755=CARTESIAN_POINT('Ctrl Pts',(-6.17419546746325,-0.290827781409624,
4.59779418863358));
#11756=CARTESIAN_POINT('Ctrl Pts',(-6.14711949228446,0.192830647320786,
4.61585919422455));
#11757=CARTESIAN_POINT('Ctrl Pts',(-6.38122030015602,0.616213166166492,
4.63390107931286));
#11758=CARTESIAN_POINT('Ctrl Pts',(-6.80413193263285,0.849857078671816,
4.65191953970996));
#11759=CARTESIAN_POINT('Ctrl Pts',(-7.28591355768388,0.822695751647876,
4.66991429633147));
#11760=CARTESIAN_POINT('Ctrl Pts',(-7.67882113931455,0.543798193542044,
4.68788504608153));
#11761=CARTESIAN_POINT('Ctrl Pts',(-7.86298344539143,0.0990860698837288,
4.70583158256722));
#11762=CARTESIAN_POINT('Ctrl Pts',(-7.79562977646068,-0.295585883755131,
4.72076651863455));
#11763=CARTESIAN_POINT('Ctrl Pts',(-7.62259402545982,-0.553684972592025,
4.73270226063253));
#11764=CARTESIAN_POINT('Ctrl Pts',(-7.38563136562569,-0.754371890467876,
4.74462971241004));
#11765=CARTESIAN_POINT('Ctrl Pts',(-7.00200477988192,-0.865035088308813,
4.75952323795895));
#11766=CARTESIAN_POINT('Ctrl Pts',(-6.54208755381532,-0.73237927966396,
4.77737036348736));
#11767=CARTESIAN_POINT('Ctrl Pts',(-6.2237590976575,-0.376028323754344,
4.7951920545367));
#11768=CARTESIAN_POINT('Ctrl Pts',(-6.14390675955708,0.0944571090275195,
4.81298816916304));
#11769=CARTESIAN_POINT('Ctrl Pts',(-6.32635880476601,0.534640108883085,
4.83075849956042));
#11770=CARTESIAN_POINT('Ctrl Pts',(-6.71446788666468,0.809896714068275,
4.84850288731427));
#11771=CARTESIAN_POINT('Ctrl Pts',(-7.18884402106963,0.83642032971082,4.86622116373149));
#11772=CARTESIAN_POINT('Ctrl Pts',(-7.6040077565224,0.606854467278431,4.88391319648774));
#11773=CARTESIAN_POINT('Ctrl Pts',(-7.83307416457905,0.192166517804397,
4.90157882330678));
#11774=CARTESIAN_POINT('Ctrl Pts',(-7.80644295598691,-0.280031406976875,
4.91921798059982));
#11775=CARTESIAN_POINT('Ctrl Pts',(-7.53313346814401,-0.665323716801619,
4.93683042576433));
#11776=CARTESIAN_POINT('Ctrl Pts',(-7.0973521810726,-0.845395310573347,
4.95441634803877));
#11777=CARTESIAN_POINT('Ctrl Pts',(-6.63325877718377,-0.76671280820668,
4.97197505561031));
#11778=CARTESIAN_POINT('Ctrl Pts',(-6.28278420709442,-0.453044306679936,
4.98950772058579));
#11779=CARTESIAN_POINT('Ctrl Pts',(-6.19628963467771,-0.152979186566042,
5.00117676314781));
#11780=CARTESIAN_POINT('Ctrl Pts',(-6.19626935608997,-0.00220549038420499,
5.00700843180463));
#11781=CARTESIAN_POINT('Ctrl Pts',(-6.2248547744189,-0.00199943343782885,
1.1016075197803));
#11782=CARTESIAN_POINT('Ctrl Pts',(-6.2248743310293,0.143406873091139,1.10723158692092));
#11783=CARTESIAN_POINT('Ctrl Pts',(-6.30828836165333,0.432372070079823,
1.11847000135813));
#11784=CARTESIAN_POINT('Ctrl Pts',(-6.6449451720994,0.733412609072189,1.13530449261712));
#11785=CARTESIAN_POINT('Ctrl Pts',(-7.08929084993495,0.808561725008331,
1.15211489002863));
#11786=CARTESIAN_POINT('Ctrl Pts',(-7.50521457605639,0.636493535969788,
1.16890177394572));
#11787=CARTESIAN_POINT('Ctrl Pts',(-7.76520183847965,0.269661650219744,
1.18566492040252));
#11788=CARTESIAN_POINT('Ctrl Pts',(-7.79029164728548,-0.178500460126232,
1.20240537393246));
#11789=CARTESIAN_POINT('Ctrl Pts',(-7.5733619556899,-0.570861085094046,
1.21912307461775));
#11790=CARTESIAN_POINT('Ctrl Pts',(-7.1814666343123,-0.787342248857585,
1.23581852081351));
#11791=CARTESIAN_POINT('Ctrl Pts',(-6.73511487871663,-0.762206257537691,
1.25249190232756));
#11792=CARTESIAN_POINT('Ctrl Pts',(-6.37088661927737,-0.503737190939526,
1.26914374509522));
#11793=CARTESIAN_POINT('Ctrl Pts',(-6.22894974433754,-0.160390496771507,
1.28300230726329));
#11794=CARTESIAN_POINT('Ctrl Pts',(-6.23748254588174,0.127860167140178,
1.29407912781801));
#11795=CARTESIAN_POINT('Ctrl Pts',(-6.32460268207204,0.402579634653007,
1.30514903917804));
#11796=CARTESIAN_POINT('Ctrl Pts',(-6.57145353853799,0.679010257848813,
1.31897302616244));
#11797=CARTESIAN_POINT('Ctrl Pts',(-6.99851538436538,0.801913846985834,
1.33554194147043));
#11798=CARTESIAN_POINT('Ctrl Pts',(-7.4248746680664,0.679006428406666,1.35209099258987));
#11799=CARTESIAN_POINT('Ctrl Pts',(-7.72020208132496,0.348444736414998,
1.3686207511464));
#11800=CARTESIAN_POINT('Ctrl Pts',(-7.79428470855507,-0.0880559677436623,
1.38513155285536));
#11801=CARTESIAN_POINT('Ctrl Pts',(-7.62498164492137,-0.496617735919016,
1.40162385464902));
#11802=CARTESIAN_POINT('Ctrl Pts',(-7.26465130631449,-0.752200318832177,
1.41809807629169));
#11803=CARTESIAN_POINT('Ctrl Pts',(-6.82404645473778,-0.776878229830484,
1.43455466287498));
#11804=CARTESIAN_POINT('Ctrl Pts',(-6.43824708026408,-0.563581766788353,
1.45099406485329));
#11805=CARTESIAN_POINT('Ctrl Pts',(-6.22527720772369,-0.178113937475093,
1.46741673691946));
#11806=CARTESIAN_POINT('Ctrl Pts',(-6.25000496641197,0.26114180105586,1.48382315214102));
#11807=CARTESIAN_POINT('Ctrl Pts',(-6.50439363062418,0.619572929497801,
1.50021377495522));
#11808=CARTESIAN_POINT('Ctrl Pts',(-6.91010778310017,0.787561126490409,
1.51658909691877));
#11809=CARTESIAN_POINT('Ctrl Pts',(-7.34261708720444,0.714029319530266,
1.53294958580271));
#11810=CARTESIAN_POINT('Ctrl Pts',(-7.66942871295271,0.421886680885055,
1.54929577826927));
#11811=CARTESIAN_POINT('Ctrl Pts',(-7.79060746309739,0.00107028729058553,
1.56562807006426));
#11812=CARTESIAN_POINT('Ctrl Pts',(-7.66943851128521,-0.419522152665003,
1.58194719524605));
#11813=CARTESIAN_POINT('Ctrl Pts',(-7.39764066575801,-0.662098928380482,
1.59553546104258));
#11814=CARTESIAN_POINT('Ctrl Pts',(-7.12800936410844,-0.747580149118017,
1.60640058684969));
#11815=CARTESIAN_POINT('Ctrl Pts',(-6.84533059531615,-0.75595077651127,
1.61726173262983));
#11816=CARTESIAN_POINT('Ctrl Pts',(-6.52426556122011,-0.622981447977388,
1.6302268277746));
#11817=CARTESIAN_POINT('Ctrl Pts',(-6.28241092024733,-0.303334910575114,
1.64529337928374));
#11818=CARTESIAN_POINT('Ctrl Pts',(-6.22511819857924,0.0766975317585018,
1.65974856169716));
#11819=CARTESIAN_POINT('Ctrl Pts',(-6.35654456974169,0.437774198474303,
1.67419574542797));
#11820=CARTESIAN_POINT('Ctrl Pts',(-6.64450567798582,0.691817599598452,
1.68863515213347));
#11821=CARTESIAN_POINT('Ctrl Pts',(-7.01862615778267,0.777215355234843,
1.7030672564649));
#11822=CARTESIAN_POINT('Ctrl Pts',(-7.3880631251269,0.673250361502341,1.71749234186559));
#11823=CARTESIAN_POINT('Ctrl Pts',(-7.66218237683517,0.405536292432383,
1.73191092401274));
#11824=CARTESIAN_POINT('Ctrl Pts',(-7.78852199146633,-0.00147573673230409,
1.74792521892452));
#11825=CARTESIAN_POINT('Ctrl Pts',(-7.65522108190052,-0.461991819856124,
1.76553253390028));
#11826=CARTESIAN_POINT('Ctrl Pts',(-7.23005076267344,-0.76759871495942,
1.78473130593167));
#11827=CARTESIAN_POINT('Ctrl Pts',(-6.75155429510695,-0.747274686068437,
1.80232278309724));
#11828=CARTESIAN_POINT('Ctrl Pts',(-6.40650202825669,-0.498234630744928,
1.81830900003889));
#11829=CARTESIAN_POINT('Ctrl Pts',(-6.24047280825274,-0.153939971712626,
1.83269297972554));
#11830=CARTESIAN_POINT('Ctrl Pts',(-6.25956175689153,0.228178208148652,
1.84707365028079));
#11831=CARTESIAN_POINT('Ctrl Pts',(-6.45895998733325,0.554399377254544,
1.86145136286506));
#11832=CARTESIAN_POINT('Ctrl Pts',(-6.79000787586996,0.745526894361726,
1.87582668352655));
#11833=CARTESIAN_POINT('Ctrl Pts',(-7.1722480535027,0.755164122979803,1.89019958026226));
#11834=CARTESIAN_POINT('Ctrl Pts',(-7.45546926618143,0.609639094019097,
1.90217609379266));
#11835=CARTESIAN_POINT('Ctrl Pts',(-7.619968516889,0.422826999155373,1.91175692450178));
#11836=CARTESIAN_POINT('Ctrl Pts',(-7.7337590448713,0.201469344983507,1.92133737878384));
#11837=CARTESIAN_POINT('Ctrl Pts',(-7.76555085481583,-0.115361161288046,
1.93331129725923));
#11838=CARTESIAN_POINT('Ctrl Pts',(-7.61724269656214,-0.467517024035713,
1.94768102414047));
#11839=CARTESIAN_POINT('Ctrl Pts',(-7.3184019335958,-0.705892482651842,
1.9620490369602));
#11840=CARTESIAN_POINT('Ctrl Pts',(-6.97345565893835,-0.766400777378709,
1.97522106259225));
#11841=CARTESIAN_POINT('Ctrl Pts',(-6.67002645875538,-0.684883575909834,
1.98719664580064));
#11842=CARTESIAN_POINT('Ctrl Pts',(-6.44246608826879,-0.517098553119758,
1.99797495600939));
#11843=CARTESIAN_POINT('Ctrl Pts',(-6.29209882837185,-0.277608420385701,
2.0087542076441));
#11844=CARTESIAN_POINT('Ctrl Pts',(-6.23942591483951,0.000274968281026084,
2.01953435056931));
#11845=CARTESIAN_POINT('Ctrl Pts',(-6.29209599648858,0.278086990361641,
2.03031566009411));
#11846=CARTESIAN_POINT('Ctrl Pts',(-6.44251218846467,0.517827822733974,
2.04109832171327));
#11847=CARTESIAN_POINT('Ctrl Pts',(-6.67016963267959,0.685306359896662,
2.05188242086643));
#11848=CARTESIAN_POINT('Ctrl Pts',(-7.03460845545162,0.784271696813748,
2.06626368121271));
#11849=CARTESIAN_POINT('Ctrl Pts',(-7.50934705445804,0.638539551533681,
2.08424384481427));
#11850=CARTESIAN_POINT('Ctrl Pts',(-7.80808915927313,0.121217390716024,
2.10582945567952));
#11851=CARTESIAN_POINT('Ctrl Pts',(-7.67515111918521,-0.460869941446203,
2.12742499092525));
#11852=CARTESIAN_POINT('Ctrl Pts',(-7.18151044916999,-0.797599664800736,
2.14903213853423));
#11853=CARTESIAN_POINT('Ctrl Pts',(-6.59025623160929,-0.708519309577169,
2.17065208288646));
#11854=CARTESIAN_POINT('Ctrl Pts',(-6.21717289845826,-0.240812476443051,
2.19228622491967));
#11855=CARTESIAN_POINT('Ctrl Pts',(-6.2618283572727,0.35625085518526,2.21393585669527));
#11856=CARTESIAN_POINT('Ctrl Pts',(-6.70100396959293,0.763867159272458,
2.235602305803));
#11857=CARTESIAN_POINT('Ctrl Pts',(-7.30069183224588,0.763966475773746,
2.25728686433886));
#11858=CARTESIAN_POINT('Ctrl Pts',(-7.74075874128088,0.355786355080811,
2.27899082117545));
#11859=CARTESIAN_POINT('Ctrl Pts',(-7.78576661945122,-0.243320634259026,
2.30071544320844));
#11860=CARTESIAN_POINT('Ctrl Pts',(-7.41089079459932,-0.713588286374201,
2.32246198389553));
#11861=CARTESIAN_POINT('Ctrl Pts',(-6.8155923591716,-0.803439914310088,
2.34423167566847));
#11862=CARTESIAN_POINT('Ctrl Pts',(-6.31753340638779,-0.464026266198107,
2.36602573364463));
#11863=CARTESIAN_POINT('Ctrl Pts',(-6.18312706441087,0.124235781248934,
2.38784535116155));
#11864=CARTESIAN_POINT('Ctrl Pts',(-6.48508519265119,0.647523045910538,
2.40969169944054));
#11865=CARTESIAN_POINT('Ctrl Pts',(-7.06309584210182,0.825972957887767,
2.43156593059124));
#11866=CARTESIAN_POINT('Ctrl Pts',(-7.60891342334618,0.563287329017383,
2.45346916382827));
#11867=CARTESIAN_POINT('Ctrl Pts',(-7.83065866400534,-0.00127617753292936,
2.47540251157));
#11868=CARTESIAN_POINT('Ctrl Pts',(-7.60891844338197,-0.566807923885036,
2.49736702311862));
#11869=CARTESIAN_POINT('Ctrl Pts',(-7.06088009394646,-0.830828943835411,
2.51936379410423));
#11870=CARTESIAN_POINT('Ctrl Pts',(-6.47877456758801,-0.651599257061967,
2.54139372857063));
#11871=CARTESIAN_POINT('Ctrl Pts',(-6.17330829597437,-0.122868357878831,
2.56345805540249));
#11872=CARTESIAN_POINT('Ctrl Pts',(-6.28698448117334,0.372896706566128,
2.5818739530266));
#11873=CARTESIAN_POINT('Ctrl Pts',(-6.56178147714618,0.645909508994359,
2.59662532895527));
#11874=CARTESIAN_POINT('Ctrl Pts',(-6.82755959943639,0.762379250809163,
2.60769790670473));
#11875=CARTESIAN_POINT('Ctrl Pts',(-7.11823191550466,0.77309106288007,2.61877977101866));
#11876=CARTESIAN_POINT('Ctrl Pts',(-7.39283797606485,0.677141608981482,
2.62987102174684));
#11877=CARTESIAN_POINT('Ctrl Pts',(-7.61353492117917,0.487124481673172,
2.64097171794249));
#11878=CARTESIAN_POINT('Ctrl Pts',(-7.74985138987256,0.229489703988864,
2.65208210394633));
#11879=CARTESIAN_POINT('Ctrl Pts',(-7.78235878160371,-0.060347586788017,
2.66320205620807));
#11880=CARTESIAN_POINT('Ctrl Pts',(-7.69452713686875,-0.389520245766072,
2.67618710514898));
#11881=CARTESIAN_POINT('Ctrl Pts',(-7.42968251892112,-0.686854983757288,
2.69104312253098));
#11882=CARTESIAN_POINT('Ctrl Pts',(-6.9981733703996,-0.811041064637613,
2.7077785073907));
#11883=CARTESIAN_POINT('Ctrl Pts',(-6.56643864129979,-0.686766100233019,
2.7245370382011));
#11884=CARTESIAN_POINT('Ctrl Pts',(-6.26644832565199,-0.351246131845318,
2.74131877561319));
#11885=CARTESIAN_POINT('Ctrl Pts',(-6.19089673530764,0.0930086272863596,
2.75812410811431));
#11886=CARTESIAN_POINT('Ctrl Pts',(-6.3635093121898,0.509979233267529,2.77495325162342));
#11887=CARTESIAN_POINT('Ctrl Pts',(-6.73202969542257,0.771572157204226,
2.79180652369004));
#11888=CARTESIAN_POINT('Ctrl Pts',(-7.1839317338843,0.797034153014602,2.80868410758528));
#11889=CARTESIAN_POINT('Ctrl Pts',(-7.58061418049775,0.577885402976202,
2.82558639907399));
#11890=CARTESIAN_POINT('Ctrl Pts',(-7.80043251707909,0.180626646990148,
2.8425133037641));
#11891=CARTESIAN_POINT('Ctrl Pts',(-7.77473827266321,-0.273178159641957,
2.85946578653905));
#11892=CARTESIAN_POINT('Ctrl Pts',(-7.51142930934868,-0.644535621799555,
2.87644320296889));
#11893=CARTESIAN_POINT('Ctrl Pts',(-7.090247475506,-0.819107951266512,2.89344615343804));
#11894=CARTESIAN_POINT('Ctrl Pts',(-6.64007239669075,-0.742719561411661,
2.9104747934985));
#11895=CARTESIAN_POINT('Ctrl Pts',(-6.29901825762491,-0.438060207003031,
2.92752931212875));
#11896=CARTESIAN_POINT('Ctrl Pts',(-6.17213529488574,0.00202864815554152,
2.94460987011375));
#11897=CARTESIAN_POINT('Ctrl Pts',(-6.29903467328276,0.442847147807371,
2.96171662669668));
#11898=CARTESIAN_POINT('Ctrl Pts',(-6.64153900261026,0.749057273900873,
2.97884972234917));
#11899=CARTESIAN_POINT('Ctrl Pts',(-7.09515820674189,0.826230598942998,
2.99600928959219));
#11900=CARTESIAN_POINT('Ctrl Pts',(-7.52096556733847,0.649964042139717,
3.01319544553617));
#11901=CARTESIAN_POINT('Ctrl Pts',(-7.7881416295986,0.273589389598386,3.03040829701253));
#11902=CARTESIAN_POINT('Ctrl Pts',(-7.81416322471417,-0.187958462889913,
3.04764793743321));
#11903=CARTESIAN_POINT('Ctrl Pts',(-7.59029004422625,-0.593236398246943,
3.06491444690837));
#11904=CARTESIAN_POINT('Ctrl Pts',(-7.18447872363049,-0.817636398679871,
3.08220789441772));
#11905=CARTESIAN_POINT('Ctrl Pts',(-6.72075832128736,-0.791696139934339,
3.0995283347252));
#11906=CARTESIAN_POINT('Ctrl Pts',(-6.34132520469639,-0.52259858497262,
3.11687581100324));
#11907=CARTESIAN_POINT('Ctrl Pts',(-6.16294093112047,-0.0922065613935315,
3.13425035266593));
#11908=CARTESIAN_POINT('Ctrl Pts',(-6.24100252329945,0.367838376905317,
3.15165197723848));
#11909=CARTESIAN_POINT('Ctrl Pts',(-6.55234143603862,0.716379447785238,
3.16908068867878));
#11910=CARTESIAN_POINT('Ctrl Pts',(-7.0020918463353,0.846056103485526,3.18653647882978));
#11911=CARTESIAN_POINT('Ctrl Pts',(-7.45259514550158,0.716373955203891,
3.20401932609763));
#11912=CARTESIAN_POINT('Ctrl Pts',(-7.76553445013922,0.366346675369135,
3.22152919662609));
#11913=CARTESIAN_POINT('Ctrl Pts',(-7.84440291089243,-0.0972364168705279,
3.23906604346409));
#11914=CARTESIAN_POINT('Ctrl Pts',(-7.66426531187148,-0.532390368454461,
3.25662980727804));
#11915=CARTESIAN_POINT('Ctrl Pts',(-7.27963605235025,-0.805423137096165,
3.27422041570518));
#11916=CARTESIAN_POINT('Ctrl Pts',(-6.80798248464413,-0.832011638635212,
3.29183778378752));
#11917=CARTESIAN_POINT('Ctrl Pts',(-6.39385226051638,-0.603245168153667,
3.30948181447676));
#11918=CARTESIAN_POINT('Ctrl Pts',(-6.16456258923952,-0.188589753805594,
3.32715239846137));
#11919=CARTESIAN_POINT('Ctrl Pts',(-6.19107396991504,0.285201839732527,
3.34484941106767));
#11920=CARTESIAN_POINT('Ctrl Pts',(-6.46598763617319,0.672844381049206,
3.36257272475332));
#11921=CARTESIAN_POINT('Ctrl Pts',(-6.90568126453254,0.855061730521347,
3.3803221784867));
#11922=CARTESIAN_POINT('Ctrl Pts',(-7.37554004917386,0.775319482500417,
3.39809764885156));
#11923=CARTESIAN_POINT('Ctrl Pts',(-7.7316309447337,0.457299820367578,3.4158988892878));
#11924=CARTESIAN_POINT('Ctrl Pts',(-7.84174000603609,0.0745662310640038,
3.43075473309166));
#11925=CARTESIAN_POINT('Ctrl Pts',(-7.79800365863135,-0.232056476805671,
3.44265191712469));
#11926=CARTESIAN_POINT('Ctrl Pts',(-7.67182066868948,-0.515199447567559,
3.45455755275379));
#11927=CARTESIAN_POINT('Ctrl Pts',(-7.37430850860215,-0.781439283284424,
3.46945566116936));
#11928=CARTESIAN_POINT('Ctrl Pts',(-6.90072597229559,-0.862196711958034,
3.48735835153518));
#11929=CARTESIAN_POINT('Ctrl Pts',(-6.50638111259522,-0.698280648937073,
3.50329380947276));
#11930=CARTESIAN_POINT('Ctrl Pts',(-6.26771696466849,-0.420467232665984,
3.51725294127665));
#11931=CARTESIAN_POINT('Ctrl Pts',(-6.16378327673368,-0.124090742239312,
3.52922891646493));
#11932=CARTESIAN_POINT('Ctrl Pts',(-6.17563970316166,0.190145148682862,
3.541215543978));
#11933=CARTESIAN_POINT('Ctrl Pts',(-6.30136031675994,0.47862813180961,3.5532129233572));
#11934=CARTESIAN_POINT('Ctrl Pts',(-6.52415787063659,0.701300976048231,
3.5652208283079));
#11935=CARTESIAN_POINT('Ctrl Pts',(-6.81305446865538,0.827485478120808,
3.57723931168856));
#11936=CARTESIAN_POINT('Ctrl Pts',(-7.12839417303149,0.839273074556283,
3.58926795489742));
#11937=CARTESIAN_POINT('Ctrl Pts',(-7.36023102178962,0.758149247707102,
3.59863178178537));
#11938=CARTESIAN_POINT('Ctrl Pts',(-7.5618318245833,0.624353944762267,3.60800077373871));
#11939=CARTESIAN_POINT('Ctrl Pts',(-7.75062769361495,0.416108732983249,
3.61871415916585));
#11940=CARTESIAN_POINT('Ctrl Pts',(-7.86629928772947,0.0415532963064746,
3.63345965175506));
#11941=CARTESIAN_POINT('Ctrl Pts',(-7.7779918817253,-0.39587268229449,3.65023477657817));
#11942=CARTESIAN_POINT('Ctrl Pts',(-7.46625718079828,-0.745141782522388,
3.66770107275509));
#11943=CARTESIAN_POINT('Ctrl Pts',(-6.99827607275313,-0.88002130153468,
3.68586089589016));
#11944=CARTESIAN_POINT('Ctrl Pts',(-6.52986865734608,-0.745124581336043,
3.70404217195174));
#11945=CARTESIAN_POINT('Ctrl Pts',(-6.20456394041314,-0.381273654072062,
3.7222445238637));
#11946=CARTESIAN_POINT('Ctrl Pts',(-6.12267644558823,0.100510595544224,
3.74046764828387));
#11947=CARTESIAN_POINT('Ctrl Pts',(-6.30977183326723,0.552341449898111,
3.75871108111533));
#11948=CARTESIAN_POINT('Ctrl Pts',(-6.70921301060823,0.836129267279029,
3.77697467535039));
#11949=CARTESIAN_POINT('Ctrl Pts',(-7.1441245198916,0.859984988516024,3.79322614015507));
#11950=CARTESIAN_POINT('Ctrl Pts',(-7.48623548722456,0.710359638299156,
3.80745809953178));
#11951=CARTESIAN_POINT('Ctrl Pts',(-7.71277070102754,0.48412224747983,3.81966559227767));
#11952=CARTESIAN_POINT('Ctrl Pts',(-7.84083027759801,0.190364482880831,
3.83188120516031));
#11953=CARTESIAN_POINT('Ctrl Pts',(-7.85295030253414,-0.130075942851775,
3.84410504587178));
#11954=CARTESIAN_POINT('Ctrl Pts',(-7.74691363433699,-0.43282273789263,
3.85633683595988));
#11955=CARTESIAN_POINT('Ctrl Pts',(-7.53756814795209,-0.676450487908387,
3.86857651327384));
#11956=CARTESIAN_POINT('Ctrl Pts',(-7.25358196284646,-0.825999495253873,
3.8808239163173));
#11957=CARTESIAN_POINT('Ctrl Pts',(-6.82749009436362,-0.875459457105686,
3.8971638473309));
#11958=CARTESIAN_POINT('Ctrl Pts',(-6.31840599454854,-0.631272784946072,
3.91760800377417));
#11959=CARTESIAN_POINT('Ctrl Pts',(-6.06955728718615,0.00123803732983087,
3.94216897705183));
#11960=CARTESIAN_POINT('Ctrl Pts',(-6.31819102434332,0.634074482232743,
3.96675822887569));
#11961=CARTESIAN_POINT('Ctrl Pts',(-6.9313053376154,0.929622791355819,3.99137353813945));
#11962=CARTESIAN_POINT('Ctrl Pts',(-7.58250506298981,0.728789845168479,
4.01601424493145));
#11963=CARTESIAN_POINT('Ctrl Pts',(-7.92366256220496,0.138392594622019,
4.04067889340962));
#11964=CARTESIAN_POINT('Ctrl Pts',(-7.77179568222589,-0.527662971229173,
4.06536647515298));
#11965=CARTESIAN_POINT('Ctrl Pts',(-7.27025795697357,-0.868934722949909,
4.08732996841401));
#11966=CARTESIAN_POINT('Ctrl Pts',(-6.75835124126733,-0.854544547073557,
4.10656171053866));
#11967=CARTESIAN_POINT('Ctrl Pts',(-6.37879399711334,-0.635954794669273,
4.1230547880809));
#11968=CARTESIAN_POINT('Ctrl Pts',(-6.1499093463627,-0.261266758101386,
4.13955596485591));
#11969=CARTESIAN_POINT('Ctrl Pts',(-6.12780704819221,0.177035632837681,
4.15606488283879));
#11970=CARTESIAN_POINT('Ctrl Pts',(-6.31855578375345,0.572773125836556,
4.17258104025126));
#11971=CARTESIAN_POINT('Ctrl Pts',(-6.64561065324521,0.807715171173621,
4.18772845995009));
#11972=CARTESIAN_POINT('Ctrl Pts',(-7.00069569962751,0.87468645863181,4.20150256960693));
#11973=CARTESIAN_POINT('Ctrl Pts',(-7.32033825743143,0.814344340487275,
4.21390324929584));
#11974=CARTESIAN_POINT('Ctrl Pts',(-7.59571864682914,0.641195296318534,
4.22630725980721));
#11975=CARTESIAN_POINT('Ctrl Pts',(-7.78924451820651,0.379269985559648,
4.23871461172216));
#11976=CARTESIAN_POINT('Ctrl Pts',(-7.87295367538825,0.0651494056917473,
4.25112517528242));
#11977=CARTESIAN_POINT('Ctrl Pts',(-7.82568225268596,-0.367234171521722,
4.26767616713046));
#11978=CARTESIAN_POINT('Ctrl Pts',(-7.54119300812834,-0.724025248548577,
4.28423413721587));
#11979=CARTESIAN_POINT('Ctrl Pts',(-7.1299107823301,-0.866436168146,4.30079557699508));
#11980=CARTESIAN_POINT('Ctrl Pts',(-6.80469982154594,-0.854722697198128,
4.31321922941577));
#11981=CARTESIAN_POINT('Ctrl Pts',(-6.50582530202995,-0.724153314531107,
4.32564485900137));
#11982=CARTESIAN_POINT('Ctrl Pts',(-6.27530903670794,-0.493779918883838,
4.3380724340676));
#11983=CARTESIAN_POINT('Ctrl Pts',(-6.14499807654234,-0.194895279444064,
4.35050178414795));
#11984=CARTESIAN_POINT('Ctrl Pts',(-6.1326836203633,0.130969847315759,4.36293259153097));
#11985=CARTESIAN_POINT('Ctrl Pts',(-6.24054332790336,0.438658395770793,
4.37536497831168));
#11986=CARTESIAN_POINT('Ctrl Pts',(-6.48850361176595,0.727358100762058,
4.38987036538262));
#11987=CARTESIAN_POINT('Ctrl Pts',(-6.89878519788956,0.898005260436416,
4.40645053432791));
#11988=CARTESIAN_POINT('Ctrl Pts',(-7.39214301970602,0.81394727492655,4.42510540352934));
#11989=CARTESIAN_POINT('Ctrl Pts',(-7.7650364742413,0.480739139420634,4.44376113789487));
#11990=CARTESIAN_POINT('Ctrl Pts',(-7.90357160220274,-3.623103406608E-6,
4.46241753166182));
#11991=CARTESIAN_POINT('Ctrl Pts',(-7.765072064783,-0.48066867355125,4.48107386788255));
#11992=CARTESIAN_POINT('Ctrl Pts',(-7.39209692797424,-0.813999851714318,
4.49972963764179));
#11993=CARTESIAN_POINT('Ctrl Pts',(-6.89897204270138,-0.897777064686935,
4.51838423828675));
#11994=CARTESIAN_POINT('Ctrl Pts',(-6.43690579425127,-0.706377273901182,
4.53703710208272));
#11995=CARTESIAN_POINT('Ctrl Pts',(-6.14753182130078,-0.29852635300287,
4.55568763786335));
#11996=CARTESIAN_POINT('Ctrl Pts',(-6.11950670544268,0.200690311117515,
4.57433527397971));
#11997=CARTESIAN_POINT('Ctrl Pts',(-6.36133752232976,0.638212076438947,
4.59297941498749));
#11998=CARTESIAN_POINT('Ctrl Pts',(-6.79877170304226,0.879965848122953,
4.6116195104013));
#11999=CARTESIAN_POINT('Ctrl Pts',(-7.29767685928348,0.851914437330659,
4.63025492201343));
#12000=CARTESIAN_POINT('Ctrl Pts',(-7.70501759766691,0.562861344844633,
4.64888520633693));
#12001=CARTESIAN_POINT('Ctrl Pts',(-7.89619288084634,0.101410721742439,
4.66750951337591));
#12002=CARTESIAN_POINT('Ctrl Pts',(-7.82628685314434,-0.308577267495686,
4.68302485728523));
#12003=CARTESIAN_POINT('Ctrl Pts',(-7.64641803457992,-0.576889867652478,
4.69543289868442));
#12004=CARTESIAN_POINT('Ctrl Pts',(-7.39997233303158,-0.785623378939254,
4.7078385298175));
#12005=CARTESIAN_POINT('Ctrl Pts',(-7.00068720444936,-0.900862697549362,
4.72334181510526));
#12006=CARTESIAN_POINT('Ctrl Pts',(-6.52149454897357,-0.762718702390436,
4.74193719606482));
#12007=CARTESIAN_POINT('Ctrl Pts',(-6.18946749999406,-0.391136044010536,
4.76052410820248));
#12008=CARTESIAN_POINT('Ctrl Pts',(-6.1060469913375,0.0999708129477241,
4.77910172767096));
#12009=CARTESIAN_POINT('Ctrl Pts',(-6.29661517993785,0.559908233001406,
4.79766964181958));
#12010=CARTESIAN_POINT('Ctrl Pts',(-6.70244964702483,0.847815493498755,
4.81622723951419));
#12011=CARTESIAN_POINT('Ctrl Pts',(-7.19897393950221,0.875640964323189,
4.83477405165335));
#12012=CARTESIAN_POINT('Ctrl Pts',(-7.63393210347268,0.635199165297035,
4.85330946175398));
#12013=CARTESIAN_POINT('Ctrl Pts',(-7.87415840450806,0.200428618681077,
4.87183314873462));
#12014=CARTESIAN_POINT('Ctrl Pts',(-7.8462682157887,-0.295087980091751,
4.89034419343159));
#12015=CARTESIAN_POINT('Ctrl Pts',(-7.559270479536,-0.6997578181279,4.90884305096593));
#12016=CARTESIAN_POINT('Ctrl Pts',(-7.10125854846447,-0.889082640532772,
4.9273272036816));
#12017=CARTESIAN_POINT('Ctrl Pts',(-6.61308396712537,-0.806345361743623,
4.94579808431053));
#12018=CARTESIAN_POINT('Ctrl Pts',(-6.24411722187037,-0.47624035230175,
4.96425287782899));
#12019=CARTESIAN_POINT('Ctrl Pts',(-6.15296011813682,-0.160062489926647,
4.97654946949845));
#12020=CARTESIAN_POINT('Ctrl Pts',(-6.15293876115034,-0.00127077166344464,
4.98269126153386));
#12021=CARTESIAN_POINT('Ctrl Pts',(-6.17520256096103,-0.00198708894523262,
1.10146101760312));
#12022=CARTESIAN_POINT('Ctrl Pts',(-6.17522335720648,0.152636088641731,
1.10744157754584));
#12023=CARTESIAN_POINT('Ctrl Pts',(-6.26397421604634,0.460181465931467,
1.11940264078387));
#12024=CARTESIAN_POINT('Ctrl Pts',(-6.62219829265502,0.780474598552503,
1.13731436110618));
#12025=CARTESIAN_POINT('Ctrl Pts',(-7.09502710563339,0.8604640532775,1.15520328301464));
#12026=CARTESIAN_POINT('Ctrl Pts',(-7.53761123589857,0.677356597316656,
1.17306606520991));
#12027=CARTESIAN_POINT('Ctrl Pts',(-7.81425257067584,0.287026630697464,
1.19090382222027));
#12028=CARTESIAN_POINT('Ctrl Pts',(-7.84094181593244,-0.189822561848461,
1.20871600217045));
#12029=CARTESIAN_POINT('Ctrl Pts',(-7.61013966093306,-0.607254329738822,
1.22650257068965));
#12030=CARTESIAN_POINT('Ctrl Pts',(-7.19324067176169,-0.837535007289599,
1.24426328742192));
#12031=CARTESIAN_POINT('Ctrl Pts',(-6.71848758862675,-0.81078612394349,
1.26199799446351));
#12032=CARTESIAN_POINT('Ctrl Pts',(-6.33116022346325,-0.535907604875262,
1.2797065735325));
#12033=CARTESIAN_POINT('Ctrl Pts',(-6.18026207378729,-0.170848153165099,
1.29444173805585));
#12034=CARTESIAN_POINT('Ctrl Pts',(-6.18933579538129,0.135568276904099,
1.3062167913918));
#12035=CARTESIAN_POINT('Ctrl Pts',(-6.28193796907153,0.427563933921057,
1.31798301358477));
#12036=CARTESIAN_POINT('Ctrl Pts',(-6.5442756777705,0.721311430477084,1.33267407278365));
#12037=CARTESIAN_POINT('Ctrl Pts',(-6.99797673974231,0.85185791707026,1.35027676526993));
#12038=CARTESIAN_POINT('Ctrl Pts',(-7.45077008597338,0.72130574984839,1.36785270105323));
#12039=CARTESIAN_POINT('Ctrl Pts',(-7.76428017317448,0.370353167602943,
1.38540183844591));
#12040=CARTESIAN_POINT('Ctrl Pts',(-7.84287078731736,-0.0928749009693313,
1.40292409570255));
#12041=CARTESIAN_POINT('Ctrl Pts',(-7.66325053119436,-0.526256204532712,
1.42041942701044));
#12042=CARTESIAN_POINT('Ctrl Pts',(-7.28117348427495,-0.797224750052114,
1.43788778901988));
#12043=CARTESIAN_POINT('Ctrl Pts',(-6.81422094277963,-0.823344619257912,
1.45532915596481));
#12044=CARTESIAN_POINT('Ctrl Pts',(-6.40557740007369,-0.597377670958505,
1.47274351267088));
#12045=CARTESIAN_POINT('Ctrl Pts',(-6.18014135114604,-0.189269109963645,
1.49013085807296));
#12046=CARTESIAN_POINT('Ctrl Pts',(-6.2063447813037,0.275500641446163,1.50749120271993));
#12047=CARTESIAN_POINT('Ctrl Pts',(-6.47538428641671,0.654503435576307,
1.52482457231741));
#12048=CARTESIAN_POINT('Ctrl Pts',(-6.90415993114079,0.831993637590178,
1.54213100041399));
#12049=CARTESIAN_POINT('Ctrl Pts',(-7.36093058729913,0.754291131752931,
1.55941054503198));
#12050=CARTESIAN_POINT('Ctrl Pts',(-7.70581436675896,0.445930495584409,
1.57666325226967));
#12051=CARTESIAN_POINT('Ctrl Pts',(-7.83356805338808,0.00210351736980688,
1.59388923591928));
#12052=CARTESIAN_POINT('Ctrl Pts',(-7.70582394465435,-0.441132803023751,
1.61108850297208));
#12053=CARTESIAN_POINT('Ctrl Pts',(-7.41957271786401,-0.696552747164017,
1.6253992073661));
#12054=CARTESIAN_POINT('Ctrl Pts',(-7.13580562433151,-0.786506150070278,
1.63683431952564));
#12055=CARTESIAN_POINT('Ctrl Pts',(-6.83842565990734,-0.795302935598094,
1.64826062329981));
#12056=CARTESIAN_POINT('Ctrl Pts',(-6.50087883949155,-0.655459856237676,
1.66189334009304));
#12057=CARTESIAN_POINT('Ctrl Pts',(-6.24683856091248,-0.319636583957497,
1.67772217495051));
#12058=CARTESIAN_POINT('Ctrl Pts',(-6.18673593956685,0.0792979977372244,
1.6928973583662));
#12059=CARTESIAN_POINT('Ctrl Pts',(-6.32462763406589,0.458013354632876,
1.70805202838354));
#12060=CARTESIAN_POINT('Ctrl Pts',(-6.6264499004516,0.724227994182597,1.72318637191565));
#12061=CARTESIAN_POINT('Ctrl Pts',(-7.01822731079915,0.813611152577389,
1.73830047742657));
#12062=CARTESIAN_POINT('Ctrl Pts',(-7.40474814051684,0.704789757388159,
1.75339453601228));
#12063=CARTESIAN_POINT('Ctrl Pts',(-7.69127468028525,0.424899737053255,
1.76846861925216));
#12064=CARTESIAN_POINT('Ctrl Pts',(-7.82317524134296,-0.000214256054242891,
1.78519536337412));
#12065=CARTESIAN_POINT('Ctrl Pts',(-7.68400292544061,-0.480657578694496,
1.80356687214843));
#12066=CARTESIAN_POINT('Ctrl Pts',(-7.24089307934962,-0.799010630883542,
1.82357396776757));
#12067=CARTESIAN_POINT('Ctrl Pts',(-6.74293367382506,-0.777755869248963,
1.84188239224313));
#12068=CARTESIAN_POINT('Ctrl Pts',(-6.38428160300257,-0.518827919852002,
1.8585022780832));
#12069=CARTESIAN_POINT('Ctrl Pts',(-6.21190652336758,-0.161263271843629,
1.87344136056984));
#12070=CARTESIAN_POINT('Ctrl Pts',(-6.23176145956434,0.235155052909281,
1.88836189008528));
#12071=CARTESIAN_POINT('Ctrl Pts',(-6.43845468102026,0.573210094242605,
1.90326411778669));
#12072=CARTESIAN_POINT('Ctrl Pts',(-6.78120758623466,0.771036152968419,
1.91814814537143));
#12073=CARTESIAN_POINT('Ctrl Pts',(-7.17651986260646,0.780947526175952,
1.93301451057625));
#12074=CARTESIAN_POINT('Ctrl Pts',(-7.4690838087241,0.6305742769914,1.94538806622837));
#12075=CARTESIAN_POINT('Ctrl Pts',(-7.63887158061852,0.43774021307995,1.95527801683068));
#12076=CARTESIAN_POINT('Ctrl Pts',(-7.75625455717709,0.209372765981586,
1.96516220579056));
#12077=CARTESIAN_POINT('Ctrl Pts',(-7.78897772922025,-0.117235198065406,
1.97750752002541));
#12078=CARTESIAN_POINT('Ctrl Pts',(-7.63621849985398,-0.479805178484218,
1.99230385729475));
#12079=CARTESIAN_POINT('Ctrl Pts',(-7.3288106015314,-0.724940155926844,
2.00708477487171));
#12080=CARTESIAN_POINT('Ctrl Pts',(-6.97443057853455,-0.787047878698219,
2.02061813346151));
#12081=CARTESIAN_POINT('Ctrl Pts',(-6.663036910551,-0.703366340083497,2.03290903791219));
#12082=CARTESIAN_POINT('Ctrl Pts',(-6.429713249652,-0.531296785721741,2.04396215844239));
#12083=CARTESIAN_POINT('Ctrl Pts',(-6.27568069467376,-0.285929863314846,
2.05500628203848));
#12084=CARTESIAN_POINT('Ctrl Pts',(-6.22179379652821,-0.00148447165528299,
2.06604174225271));
#12085=CARTESIAN_POINT('Ctrl Pts',(-6.27567723842726,0.282625283926166,
2.0770685423675));
#12086=CARTESIAN_POINT('Ctrl Pts',(-6.42939321834636,0.527569244817696,
2.08808682846216));
#12087=CARTESIAN_POINT('Ctrl Pts',(-6.66180436480139,0.698523534700444,
2.09909676470742));
#12088=CARTESIAN_POINT('Ctrl Pts',(-7.03352012631891,0.799423308390042,
2.11376548571774));
#12089=CARTESIAN_POINT('Ctrl Pts',(-7.51702000256108,0.650830743926028,
2.13208194275696));
#12090=CARTESIAN_POINT('Ctrl Pts',(-7.8205544699971,0.12477872778957,2.15402963008721));
#12091=CARTESIAN_POINT('Ctrl Pts',(-7.68544758554438,-0.465859683502365,
2.17594706678624));
#12092=CARTESIAN_POINT('Ctrl Pts',(-7.18532832918539,-0.806749907827285,
2.19783506274917));
#12093=CARTESIAN_POINT('Ctrl Pts',(-6.58761900266066,-0.716477849063796,
2.21969487371389));
#12094=CARTESIAN_POINT('Ctrl Pts',(-6.21132525852498,-0.244398599379355,
2.24152759150295));
#12095=CARTESIAN_POINT('Ctrl Pts',(-6.2565166557362,0.3569122874933,2.26333440391098));
#12096=CARTESIAN_POINT('Ctrl Pts',(-6.69813227966462,0.766495972123007,
2.2851164884739));
#12097=CARTESIAN_POINT('Ctrl Pts',(-7.29979559743913,0.766377681005144,
2.30687505361852));
#12098=CARTESIAN_POINT('Ctrl Pts',(-7.7403172038414,0.357478557881761,2.32861132352834));
#12099=CARTESIAN_POINT('Ctrl Pts',(-7.78508314321668,-0.241314211311507,
2.35032654112574));
#12100=CARTESIAN_POINT('Ctrl Pts',(-7.41096299128847,-0.710285258646494,
2.37202196782575));
#12101=CARTESIAN_POINT('Ctrl Pts',(-6.81823980426185,-0.799529018877506,
2.39369887989847));
#12102=CARTESIAN_POINT('Ctrl Pts',(-6.32343193216603,-0.462069625636124,
2.41535857127149));
#12103=CARTESIAN_POINT('Ctrl Pts',(-6.19033403334486,0.121430361598332,
2.43700234837564));
#12104=CARTESIAN_POINT('Ctrl Pts',(-6.48944013553029,0.639347819738511,
2.45863153303831));
#12105=CARTESIAN_POINT('Ctrl Pts',(-7.06062039853485,0.815467008999971,
2.48024745795251));
#12106=CARTESIAN_POINT('Ctrl Pts',(-7.59882665791512,0.556211166886447,
2.50185147160134));
#12107=CARTESIAN_POINT('Ctrl Pts',(-7.81691597971047,0.00038587243355178,
2.52344492141857));
#12108=CARTESIAN_POINT('Ctrl Pts',(-7.59884810631217,-0.555213231600651,
2.5450292014295));
#12109=CARTESIAN_POINT('Ctrl Pts',(-7.06125744429576,-0.813974168132374,
2.56660562283359));
#12110=CARTESIAN_POINT('Ctrl Pts',(-6.49143383198293,-0.638312378386942,
2.58817573968482));
#12111=CARTESIAN_POINT('Ctrl Pts',(-6.19309159486605,-0.121506544825599,
2.60974057380503));
#12112=CARTESIAN_POINT('Ctrl Pts',(-6.30414628890434,0.362095563250968,
2.62770881360045));
#12113=CARTESIAN_POINT('Ctrl Pts',(-6.57188215917242,0.628050171743863,
2.64208135096746));
#12114=CARTESIAN_POINT('Ctrl Pts',(-6.83060733093959,0.741402467988298,
2.65286053512832));
#12115=CARTESIAN_POINT('Ctrl Pts',(-7.11331019485116,0.751800822313028,
2.66363943998543));
#12116=CARTESIAN_POINT('Ctrl Pts',(-7.38015321254041,0.658536578249394,
2.67441829878632));
#12117=CARTESIAN_POINT('Ctrl Pts',(-7.59442540813206,0.474028701024785,
2.68519731735848));
#12118=CARTESIAN_POINT('Ctrl Pts',(-7.72664835318823,0.224078813661572,
2.69597649059435));
#12119=CARTESIAN_POINT('Ctrl Pts',(-7.75814251512839,-0.0568684122326128,
2.7067563322709));
#12120=CARTESIAN_POINT('Ctrl Pts',(-7.67305026831101,-0.375670601170515,
2.71933299465532));
#12121=CARTESIAN_POINT('Ctrl Pts',(-7.41675242429056,-0.663319154262185,
2.73370861079294));
#12122=CARTESIAN_POINT('Ctrl Pts',(-6.99972126318494,-0.783265764622907,
2.74988403280801));
#12123=CARTESIAN_POINT('Ctrl Pts',(-6.58300990508826,-0.663244925260623,
2.76606207030967));
#12124=CARTESIAN_POINT('Ctrl Pts',(-6.29383153821051,-0.339717208918772,
2.78224374459041));
#12125=CARTESIAN_POINT('Ctrl Pts',(-6.22114054700406,0.0881212098583566,
2.79842947681081));
#12126=CARTESIAN_POINT('Ctrl Pts',(-6.38724602124502,0.489197356400545,
2.81461997314655));
#12127=CARTESIAN_POINT('Ctrl Pts',(-6.74139139837251,0.740504683130387,
2.83081572177923));
#12128=CARTESIAN_POINT('Ctrl Pts',(-7.17515482616827,0.76487797258106,2.84701748262569));
#12129=CARTESIAN_POINT('Ctrl Pts',(-7.55548063740019,0.554694931751024,
2.86322547779102));
#12130=CARTESIAN_POINT('Ctrl Pts',(-7.76598006770104,0.174143761765996,
2.87944106971308));
#12131=CARTESIAN_POINT('Ctrl Pts',(-7.74133660602088,-0.260082341241471,
2.89566309355239));
#12132=CARTESIAN_POINT('Ctrl Pts',(-7.48957685241318,-0.615046118600353,
2.91189415966483));
#12133=CARTESIAN_POINT('Ctrl Pts',(-7.08731533016645,-0.781714319571146,
2.92813385307331));
#12134=CARTESIAN_POINT('Ctrl Pts',(-6.65779777358391,-0.70877510401241,
2.94438283541206));
#12135=CARTESIAN_POINT('Ctrl Pts',(-6.33271975622983,-0.418314727228539,
2.96064163431084));
#12136=CARTESIAN_POINT('Ctrl Pts',(-6.21192448996774,0.000848146316009892,
2.97691080417122));
#12137=CARTESIAN_POINT('Ctrl Pts',(-6.33273084797174,0.420316475281392,
2.99319088962537));
#12138=CARTESIAN_POINT('Ctrl Pts',(-6.65841919119061,0.711426102093092,
3.00948242360202));
#12139=CARTESIAN_POINT('Ctrl Pts',(-7.08938365463165,0.78469653047417,3.02578593995235));
#12140=CARTESIAN_POINT('Ctrl Pts',(-7.49358481171723,0.61732386108425,3.04210195971773));
#12141=CARTESIAN_POINT('Ctrl Pts',(-7.74698795349186,0.260274136600851,
3.05843100290411));
#12142=CARTESIAN_POINT('Ctrl Pts',(-7.77161091961628,-0.177229268565413,
3.07477358371368));
#12143=CARTESIAN_POINT('Ctrl Pts',(-7.5595133072481,-0.561104620871015,
3.0911302014686));
#12144=CARTESIAN_POINT('Ctrl Pts',(-7.17535047001025,-0.773488637585987,
3.10750136160667));
#12145=CARTESIAN_POINT('Ctrl Pts',(-6.73667244369075,-0.748911461799866,
3.12388755084162));
#12146=CARTESIAN_POINT('Ctrl Pts',(-6.3779682885093,-0.494471004158721,
3.14028925748387));
#12147=CARTESIAN_POINT('Ctrl Pts',(-6.20944935172518,-0.0877920636709064,
3.15670695538732));
#12148=CARTESIAN_POINT('Ctrl Pts',(-6.28319879502128,0.346646282224702,
3.17314111625288));
#12149=CARTESIAN_POINT('Ctrl Pts',(-6.57708076320731,0.675598555420789,
3.18959220330918));
#12150=CARTESIAN_POINT('Ctrl Pts',(-7.00137860324948,0.797906523574267,
3.20606066596027));
#12151=CARTESIAN_POINT('Ctrl Pts',(-7.42617378260305,0.675596701009556,
3.22254695486609));
#12152=CARTESIAN_POINT('Ctrl Pts',(-7.72111320507981,0.345664903192319,
3.23905150388902));
#12153=CARTESIAN_POINT('Ctrl Pts',(-7.7953969119236,-0.0911079815633575,
3.25557474416723));
#12154=CARTESIAN_POINT('Ctrl Pts',(-7.62572261395765,-0.500930075649132,
3.27211709319075));
#12155=CARTESIAN_POINT('Ctrl Pts',(-7.26359060619952,-0.757969018039986,
3.28867896364162));
#12156=CARTESIAN_POINT('Ctrl Pts',(-6.8196773785154,-0.782976033006322,
3.3052607585784));
#12157=CARTESIAN_POINT('Ctrl Pts',(-6.43002407375901,-0.567712626192564,
3.32186286665882));
#12158=CARTESIAN_POINT('Ctrl Pts',(-6.2143495238102,-0.177650477030896,
3.33848567746599));
#12159=CARTESIAN_POINT('Ctrl Pts',(-6.23929452274523,0.267931676361288,
3.35512955696615));
#12160=CARTESIAN_POINT('Ctrl Pts',(-6.4977981727106,0.632417428400449,3.3717948862143));
#12161=CARTESIAN_POINT('Ctrl Pts',(-6.91116723721851,0.803716352677741,
3.38848198687104));
#12162=CARTESIAN_POINT('Ctrl Pts',(-7.35283140859241,0.728752415779589,
3.40519128182654));
#12163=CARTESIAN_POINT('Ctrl Pts',(-7.68751682991823,0.429843740878194,
3.42192294577688));
#12164=CARTESIAN_POINT('Ctrl Pts',(-7.79099865641625,0.0701396538138709,
3.43588523419587));
#12165=CARTESIAN_POINT('Ctrl Pts',(-7.74989579680847,-0.21802096983869,
3.44706617600471));
#12166=CARTESIAN_POINT('Ctrl Pts',(-7.63131205058786,-0.48411169588832,
3.45825488852589));
#12167=CARTESIAN_POINT('Ctrl Pts',(-7.35171966125215,-0.734316353658553,
3.47225592024697));
#12168=CARTESIAN_POINT('Ctrl Pts',(-6.90665634422983,-0.810213610247401,
3.48908075059773));
#12169=CARTESIAN_POINT('Ctrl Pts',(-6.53604125268008,-0.656166268075892,
3.50405734901444));
#12170=CARTESIAN_POINT('Ctrl Pts',(-6.31172510564101,-0.395058130413869,
3.51717721810318));
#12171=CARTESIAN_POINT('Ctrl Pts',(-6.21403211052705,-0.11648505246751,
3.5284338585998));
#12172=CARTESIAN_POINT('Ctrl Pts',(-6.22517418787314,0.178897331422162,
3.53970134734807));
#12173=CARTESIAN_POINT('Ctrl Pts',(-6.34335895664989,0.450096638989748,
3.55097987580857));
#12174=CARTESIAN_POINT('Ctrl Pts',(-6.55282538255646,0.659451018575483,
3.56226945063314));
#12175=CARTESIAN_POINT('Ctrl Pts',(-6.82446778576932,0.778103756403872,
3.57357018144722));
#12176=CARTESIAN_POINT('Ctrl Pts',(-7.12101306693323,0.789192713545858,
3.58488192569325));
#12177=CARTESIAN_POINT('Ctrl Pts',(-7.33906330667987,0.712896965876082,
3.59368882725176));
#12178=CARTESIAN_POINT('Ctrl Pts',(-7.52869402188939,0.58704644286916,3.60250150300269));
#12179=CARTESIAN_POINT('Ctrl Pts',(-7.70630123965848,0.391148862353906,
3.61257978479708));
#12180=CARTESIAN_POINT('Ctrl Pts',(-7.81514745185466,0.0387319382513335,
3.62645378552755));
#12181=CARTESIAN_POINT('Ctrl Pts',(-7.7320534206871,-0.372945464851778,
3.64224111773929));
#12182=CARTESIAN_POINT('Ctrl Pts',(-7.43860263654834,-0.701759159899474,
3.65868352683148));
#12183=CARTESIAN_POINT('Ctrl Pts',(-6.99790910892847,-0.828797861504417,
3.67578437922259));
#12184=CARTESIAN_POINT('Ctrl Pts',(-6.55664423613565,-0.70174357995305,
3.69291144840077));
#12185=CARTESIAN_POINT('Ctrl Pts',(-6.25005791143385,-0.358869278941272,
3.7100648670323));
#12186=CARTESIAN_POINT('Ctrl Pts',(-6.17282669341117,0.0953431157116756,
3.72724477239473));
#12187=CARTESIAN_POINT('Ctrl Pts',(-6.34926472763597,0.521516954352712,
3.74445126049261));
#12188=CARTESIAN_POINT('Ctrl Pts',(-6.72616431631433,0.789332181942143,
3.76168447228502));
#12189=CARTESIAN_POINT('Ctrl Pts',(-7.13675574522559,0.811884513458825,
3.77702664030951));
#12190=CARTESIAN_POINT('Ctrl Pts',(-7.45988117366292,0.670575550442469,
3.79046840933465));
#12191=CARTESIAN_POINT('Ctrl Pts',(-7.67392353281915,0.456831908457597,
3.80200188063455));
#12192=CARTESIAN_POINT('Ctrl Pts',(-7.79496970644638,0.179188233396773,
3.81354733579817));
#12193=CARTESIAN_POINT('Ctrl Pts',(-7.80644272472456,-0.12379090386609,
3.8251047492067));
#12194=CARTESIAN_POINT('Ctrl Pts',(-7.70615482539854,-0.410154530705009,
3.83667418041178));
#12195=CARTESIAN_POINT('Ctrl Pts',(-7.50807322282844,-0.640695822001223,
3.84825558476824));
#12196=CARTESIAN_POINT('Ctrl Pts',(-7.23924588079012,-0.782272634525382,
3.85984901862582));
#12197=CARTESIAN_POINT('Ctrl Pts',(-6.8357314622921,-0.829131775621971,
3.87532291717216));
#12198=CARTESIAN_POINT('Ctrl Pts',(-6.35327616573594,-0.59781018040019,
3.89469527550241));
#12199=CARTESIAN_POINT('Ctrl Pts',(-6.11713987966773,0.00207052637070815,
3.91799017117406));
#12200=CARTESIAN_POINT('Ctrl Pts',(-6.35307678245142,0.602907531120579,
3.94133291042122));
#12201=CARTESIAN_POINT('Ctrl Pts',(-6.93566081689883,0.883875082041324,
3.96472352664209));
#12202=CARTESIAN_POINT('Ctrl Pts',(-7.55515623959697,0.69295296286722,3.98816179669967));
#12203=CARTESIAN_POINT('Ctrl Pts',(-7.88013810709561,0.130810632835588,
4.01164757955687));
#12204=CARTESIAN_POINT('Ctrl Pts',(-7.73550042824472,-0.504166213312069,
4.03518059168276));
#12205=CARTESIAN_POINT('Ctrl Pts',(-7.25691555291904,-0.829965934756777,
4.05614067290557));
#12206=CARTESIAN_POINT('Ctrl Pts',(-6.76789466611817,-0.816273162480241,
4.07451081161441));
#12207=CARTESIAN_POINT('Ctrl Pts',(-6.40500652557533,-0.607330529488023,
4.09027725224445));
#12208=CARTESIAN_POINT('Ctrl Pts',(-6.18597544009142,-0.248853481949266,
4.10606432834162));
#12209=CARTESIAN_POINT('Ctrl Pts',(-6.16476183860982,0.170855301645688,
4.1218718654511));
#12210=CARTESIAN_POINT('Ctrl Pts',(-6.3475351341277,0.550140873965967,4.13769986829671));
#12211=CARTESIAN_POINT('Ctrl Pts',(-6.66120500560645,0.775526485791483,
4.15222680408194));
#12212=CARTESIAN_POINT('Ctrl Pts',(-7.00205431618851,0.839831878170417,
4.16544832658668));
#12213=CARTESIAN_POINT('Ctrl Pts',(-7.30908336124065,0.781894279466921,
4.17735870006853));
#12214=CARTESIAN_POINT('Ctrl Pts',(-7.57377766559882,0.615484497922989,
4.18928029921752));
#12215=CARTESIAN_POINT('Ctrl Pts',(-7.75993041088309,0.363580471659928,
4.20121293126314));
#12216=CARTESIAN_POINT('Ctrl Pts',(-7.84051159534739,0.0612598680482373,
4.21315653403017));
#12217=CARTESIAN_POINT('Ctrl Pts',(-7.79502050738924,-0.3551661585163,4.22909611233079));
#12218=CARTESIAN_POINT('Ctrl Pts',(-7.520840575019,-0.69919923882563,4.24505660563019));
#12219=CARTESIAN_POINT('Ctrl Pts',(-7.12391614845427,-0.836671814188821,
4.26103935959678));
#12220=CARTESIAN_POINT('Ctrl Pts',(-6.80983700920401,-0.825379971791792,
4.27303686635832));
#12221=CARTESIAN_POINT('Ctrl Pts',(-6.5209788758192,-0.699206911902937,
4.28504501164974));
#12222=CARTESIAN_POINT('Ctrl Pts',(-6.29801755032192,-0.4764180427961,4.29706359373192));
#12223=CARTESIAN_POINT('Ctrl Pts',(-6.17188017799352,-0.187148419627673,
4.3090925578342));
#12224=CARTESIAN_POINT('Ctrl Pts',(-6.15992888821969,0.128470193897301,
4.32113188034415));
#12225=CARTESIAN_POINT('Ctrl Pts',(-6.26445823392466,0.426710184996707,
4.33318130259563));
#12226=CARTESIAN_POINT('Ctrl Pts',(-6.5049581998047,0.706766049163178,4.34725107983906));
#12227=CARTESIAN_POINT('Ctrl Pts',(-6.90326744518671,0.872503536145515,
4.36334696251586));
#12228=CARTESIAN_POINT('Ctrl Pts',(-7.38281029184237,0.790877765138433,
4.38147673975636));
#12229=CARTESIAN_POINT('Ctrl Pts',(-7.74572176421123,0.466691558041768,
4.39962862353129));
#12230=CARTESIAN_POINT('Ctrl Pts',(-7.88075906451644,-0.00163370218810728,
4.41780197870862));
#12231=CARTESIAN_POINT('Ctrl Pts',(-7.74575034874242,-0.470472473332599,
4.4359965458689));
#12232=CARTESIAN_POINT('Ctrl Pts',(-7.38159674501435,-0.796028387119033,
4.45421188622969));
#12233=CARTESIAN_POINT('Ctrl Pts',(-6.89950908277415,-0.878014102013699,
4.47244763868539));
#12234=CARTESIAN_POINT('Ctrl Pts',(-6.44720261643851,-0.690747124710534,
4.49070339435891));
#12235=CARTESIAN_POINT('Ctrl Pts',(-6.1635529610742,-0.291109214224599,
4.50897875507623));
#12236=CARTESIAN_POINT('Ctrl Pts',(-6.13597125160479,0.198699563497598,
4.52727330335656));
#12237=CARTESIAN_POINT('Ctrl Pts',(-6.37346031508276,0.628542467914837,
4.54558662808959));
#12238=CARTESIAN_POINT('Ctrl Pts',(-6.80365868518738,0.866395911895694,
4.56391827748347));
#12239=CARTESIAN_POINT('Ctrl Pts',(-7.29496543480093,0.838858349286866,
4.58226786138585));
#12240=CARTESIAN_POINT('Ctrl Pts',(-7.69664252566589,0.553931788000972,
4.60063481598526));
#12241=CARTESIAN_POINT('Ctrl Pts',(-7.88544935552637,0.0984229027900429,
4.61901894616799));
#12242=CARTESIAN_POINT('Ctrl Pts',(-7.81642268275138,-0.306825472701288,
4.63435246271745));
#12243=CARTESIAN_POINT('Ctrl Pts',(-7.6384752345081,-0.572297394360716,
4.64662804193218));
#12244=CARTESIAN_POINT('Ctrl Pts',(-7.39450780779738,-0.778951033732389,
4.6589089055924));
#12245=CARTESIAN_POINT('Ctrl Pts',(-6.99888600622643,-0.893209786912865,
4.67426881313452));
#12246=CARTESIAN_POINT('Ctrl Pts',(-6.52343435780138,-0.756238112350475,
4.69271630273848));
#12247=CARTESIAN_POINT('Ctrl Pts',(-6.19353907010138,-0.38716921999977,
4.71117825554814));
#12248=CARTESIAN_POINT('Ctrl Pts',(-6.11047969071254,0.101292654240927,
4.72965444234953));
#12249=CARTESIAN_POINT('Ctrl Pts',(-6.30018765284877,0.559379591273636,
4.7481442280249));
#12250=CARTESIAN_POINT('Ctrl Pts',(-6.70482157814926,0.846542371924633,
4.76664715301658));
#12251=CARTESIAN_POINT('Ctrl Pts',(-7.20056270996627,0.874413303374147,
4.78516266216818));
#12252=CARTESIAN_POINT('Ctrl Pts',(-7.63543291420515,0.634124121998299,
4.80369025418887));
#12253=CARTESIAN_POINT('Ctrl Pts',(-7.87597488452673,0.198982319936917,
4.8222293469264));
#12254=CARTESIAN_POINT('Ctrl Pts',(-7.84811680670301,-0.297641763084105,
4.8407794771796));
#12255=CARTESIAN_POINT('Ctrl Pts',(-7.5602099822393,-0.703770114540898,
4.85933989842883));
#12256=CARTESIAN_POINT('Ctrl Pts',(-7.10005207809272,-0.894083431664867,
4.87791045675167));
#12257=CARTESIAN_POINT('Ctrl Pts',(-6.60892470845569,-0.810928286707249,
4.89649198113447));
#12258=CARTESIAN_POINT('Ctrl Pts',(-6.23721493477519,-0.478496418619897,
4.91507955704552));
#12259=CARTESIAN_POINT('Ctrl Pts',(-6.14524645745769,-0.1595934132457,4.92748136616133));
#12260=CARTESIAN_POINT('Ctrl Pts',(-6.14522490872935,0.000623928402563829,
4.93367829887062));
#12261=CARTESIAN_POINT('Ctrl Pts',(-6.14410050409056,-0.00048591577833035,
1.06275739095565));
#12262=CARTESIAN_POINT('Ctrl Pts',(-6.14412207724039,0.159913661349453,
1.06896137214896));
#12263=CARTESIAN_POINT('Ctrl Pts',(-6.23622929144067,0.47922381214816,1.08138051738368));
#12264=CARTESIAN_POINT('Ctrl Pts',(-6.60844007459979,0.8121004889077,1.09999411362412));
#12265=CARTESIAN_POINT('Ctrl Pts',(-7.1002710567507,0.895387320978274,1.11860340208149));
#12266=CARTESIAN_POINT('Ctrl Pts',(-7.56113081871182,0.704794039986598,
1.13720366503272));
#12267=CARTESIAN_POINT('Ctrl Pts',(-7.84953105077671,0.29801802119025,1.15579741148642));
#12268=CARTESIAN_POINT('Ctrl Pts',(-7.87744617007159,-0.199444272232843,
1.17438121295457));
#12269=CARTESIAN_POINT('Ctrl Pts',(-7.63650373307356,-0.635363371911168,
1.192955922617));
#12270=CARTESIAN_POINT('Ctrl Pts',(-7.20080576831759,-0.876103765907077,
1.21152037655879));
#12271=CARTESIAN_POINT('Ctrl Pts',(-6.70415725883354,-0.848183653696337,
1.23007445249145));
#12272=CARTESIAN_POINT('Ctrl Pts',(-6.29857446753047,-0.560427267789544,
1.24861722602105));
#12273=CARTESIAN_POINT('Ctrl Pts',(-6.14039323611512,-0.177880372686661,
1.26406029904333));
#12274=CARTESIAN_POINT('Ctrl Pts',(-6.14989802726945,0.143427644563409,
1.2764078954173));
#12275=CARTESIAN_POINT('Ctrl Pts',(-6.2470304684292,0.449740527003316,1.2887513666884));
#12276=CARTESIAN_POINT('Ctrl Pts',(-6.52237137413574,0.75811907727139,1.3041737332961));
#12277=CARTESIAN_POINT('Ctrl Pts',(-6.99898578295027,0.895317551226051,
1.3226669278757));
#12278=CARTESIAN_POINT('Ctrl Pts',(-7.47505081224439,0.758114363165164,
1.34114661424288));
#12279=CARTESIAN_POINT('Ctrl Pts',(-7.80495431777145,0.388892460514594,
1.35961201601459));
#12280=CARTESIAN_POINT('Ctrl Pts',(-7.88775781679195,-0.0988491436399237,
1.37806276650224));
#12281=CARTESIAN_POINT('Ctrl Pts',(-7.69854028573051,-0.555520196691456,
1.39649832149178));
#12282=CARTESIAN_POINT('Ctrl Pts',(-7.29569627612792,-0.841277260574458,
1.41491822157768));
#12283=CARTESIAN_POINT('Ctrl Pts',(-6.80299959078561,-0.86888494277178,
1.43332198328018));
#12284=CARTESIAN_POINT('Ctrl Pts',(-6.37152153031215,-0.630343777158989,
1.4517091401951));
#12285=CARTESIAN_POINT('Ctrl Pts',(-6.13331261235062,-0.199204052893853,
1.47007923391518));
#12286=CARTESIAN_POINT('Ctrl Pts',(-6.16097031239077,0.29211742748464,1.4884318061235));
#12287=CARTESIAN_POINT('Ctrl Pts',(-6.44550960543965,0.693025905897973,
1.50676641948554));
#12288=CARTESIAN_POINT('Ctrl Pts',(-6.89927742024254,0.880903934890723,
1.52508263139204));
#12289=CARTESIAN_POINT('Ctrl Pts',(-7.38295020622619,0.79866296575333,1.54338002563818));
#12290=CARTESIAN_POINT('Ctrl Pts',(-7.74834974407646,0.472007046947655,
1.56165816198871));
#12291=CARTESIAN_POINT('Ctrl Pts',(-7.88379136539645,0.0015932228150884,
1.57991668890152));
#12292=CARTESIAN_POINT('Ctrl Pts',(-7.74836207707285,-0.468425528948212,
1.59815508413406));
#12293=CARTESIAN_POINT('Ctrl Pts',(-7.44470643423547,-0.739409180084324,
1.61333689773705));
#12294=CARTESIAN_POINT('Ctrl Pts',(-7.14358065498685,-0.83487032164026,
1.62547158256094));
#12295=CARTESIAN_POINT('Ctrl Pts',(-6.82794859576551,-0.84421204181463,
1.63759925840241));
#12296=CARTESIAN_POINT('Ctrl Pts',(-6.46957391377044,-0.695762871566993,
1.65207286856862));
#12297=CARTESIAN_POINT('Ctrl Pts',(-6.19976126317667,-0.339120077397132,
1.66888349074963));
#12298=CARTESIAN_POINT('Ctrl Pts',(-6.13589629964516,0.0846784598942406,
1.68500450708744));
#12299=CARTESIAN_POINT('Ctrl Pts',(-6.2824074133963,0.487111860626291,1.70110795274312));
#12300=CARTESIAN_POINT('Ctrl Pts',(-6.60319657410942,0.770074716109897,
1.71719366153553));
#12301=CARTESIAN_POINT('Ctrl Pts',(-7.01969476173132,0.865111288516179,
1.73326137514033));
#12302=CARTESIAN_POINT('Ctrl Pts',(-7.4306928078077,0.749411346956209,1.74931089435423));
#12303=CARTESIAN_POINT('Ctrl Pts',(-7.7354220185315,0.45175405795709,1.76534199326832));
#12304=CARTESIAN_POINT('Ctrl Pts',(-7.87573129698657,-0.000424291859933977,
1.78313350574046));
#12305=CARTESIAN_POINT('Ctrl Pts',(-7.72768926849582,-0.5115400388969,1.8026773859338));
#12306=CARTESIAN_POINT('Ctrl Pts',(-7.25623748727849,-0.850272059219606,
1.82396401709854));
#12307=CARTESIAN_POINT('Ctrl Pts',(-6.72636750519522,-0.82766223357698,
1.84344526759864));
#12308=CARTESIAN_POINT('Ctrl Pts',(-6.34471506576865,-0.552133547071731,
1.86113015122148));
#12309=CARTESIAN_POINT('Ctrl Pts',(-6.16128171743482,-0.171634315548159,
1.87702681595704));
#12310=CARTESIAN_POINT('Ctrl Pts',(-6.18240969119849,0.250208795734504,
1.89290359619399));
#12311=CARTESIAN_POINT('Ctrl Pts',(-6.40235309302082,0.609934372469904,
1.90876032957526));
#12312=CARTESIAN_POINT('Ctrl Pts',(-6.76705946071901,0.820428504223453,
1.92459690112763));
#12313=CARTESIAN_POINT('Ctrl Pts',(-7.18765603844751,0.830971128018649,
1.94041310898236));
#12314=CARTESIAN_POINT('Ctrl Pts',(-7.49890147790259,0.670990327777045,
1.95357632534897));
#12315=CARTESIAN_POINT('Ctrl Pts',(-7.67951671280284,0.465859266917597,
1.96409665265068));
#12316=CARTESIAN_POINT('Ctrl Pts',(-7.8043767947787,0.222944738654196,1.97461011272258));
#12317=CARTESIAN_POINT('Ctrl Pts',(-7.83917648143533,-0.124419817932346,
1.98773878468873));
#12318=CARTESIAN_POINT('Ctrl Pts',(-7.67672672626751,-0.509974597233562,
2.00347273819115));
#12319=CARTESIAN_POINT('Ctrl Pts',(-7.34990055604162,-0.770583214113921,
2.01918541233071));
#12320=CARTESIAN_POINT('Ctrl Pts',(-6.97321369524517,-0.836592625313303,
2.03356972932625));
#12321=CARTESIAN_POINT('Ctrl Pts',(-6.64228894118503,-0.747654759769428,
2.04663120532969));
#12322=CARTESIAN_POINT('Ctrl Pts',(-6.39438122166063,-0.564827652399831,
2.05837453042368));
#12323=CARTESIAN_POINT('Ctrl Pts',(-6.23076075497057,-0.304172929347532,
2.07010604415484));
#12324=CARTESIAN_POINT('Ctrl Pts',(-6.17353255087278,-0.00207671493773103,
2.08182557707505));
#12325=CARTESIAN_POINT('Ctrl Pts',(-6.23075516145379,0.299589335459152,
2.09353321005446));
#12326=CARTESIAN_POINT('Ctrl Pts',(-6.39393436245754,0.55960479989559,2.10522886005712));
#12327=CARTESIAN_POINT('Ctrl Pts',(-6.64058776547682,0.741023493503706,
2.11691253477686));
#12328=CARTESIAN_POINT('Ctrl Pts',(-7.03497389811195,0.848068440992084,
2.13247484644387));
#12329=CARTESIAN_POINT('Ctrl Pts',(-7.54770624434186,0.690428321903564,
2.15189724253272));
#12330=CARTESIAN_POINT('Ctrl Pts',(-7.86933514613633,0.132858902880382,
2.17515629625777));
#12331=CARTESIAN_POINT('Ctrl Pts',(-7.72615768132878,-0.492675738532521,
2.19836709561093));
#12332=CARTESIAN_POINT('Ctrl Pts',(-7.19681213796589,-0.853377790664305,
2.2215297913067));
#12333=CARTESIAN_POINT('Ctrl Pts',(-6.56474624880106,-0.75781946082691,
2.24464435055119));
#12334=CARTESIAN_POINT('Ctrl Pts',(-6.16722750860373,-0.258948675165486,
2.26771088327184));
#12335=CARTESIAN_POINT('Ctrl Pts',(-6.2150427332084,0.37583414834438,2.29072949788041));
#12336=CARTESIAN_POINT('Ctrl Pts',(-6.68088653563404,0.807733315243065,
2.31370036331483));
#12337=CARTESIAN_POINT('Ctrl Pts',(-7.31482602441585,0.807489047368646,
2.3366236806125));
#12338=CARTESIAN_POINT('Ctrl Pts',(-7.77841287257781,0.377009500959829,
2.35949969509982));
#12339=CARTESIAN_POINT('Ctrl Pts',(-7.82534987879143,-0.252577161845689,
2.38232869014123));
#12340=CARTESIAN_POINT('Ctrl Pts',(-7.43233507498677,-0.745015046067986,
2.40511098975844));
#12341=CARTESIAN_POINT('Ctrl Pts',(-6.81055800597004,-0.838490467640577,
2.42784695662596));
#12342=CARTESIAN_POINT('Ctrl Pts',(-6.29223116029819,-0.484813997427444,
2.45053699256128));
#12343=CARTESIAN_POINT('Ctrl Pts',(-6.15310912579615,0.125775995325234,
2.47318153832518));
#12344=CARTESIAN_POINT('Ctrl Pts',(-6.46580906475682,0.666919744066789,
2.4957810706093));
#12345=CARTESIAN_POINT('Ctrl Pts',(-7.06192948798325,0.850560608805366,
2.51833610880894));
#12346=CARTESIAN_POINT('Ctrl Pts',(-7.62273575658636,0.580234313774985,
2.540847196889));
#12347=CARTESIAN_POINT('Ctrl Pts',(-7.84952792540534,0.00176358429277413,
2.5633149405221));
#12348=CARTESIAN_POINT('Ctrl Pts',(-7.62277137533754,-0.575494391866743,
2.58573992305321));
#12349=CARTESIAN_POINT('Ctrl Pts',(-7.0649305920516,-0.84380626649313,2.60812288483676));
#12350=CARTESIAN_POINT('Ctrl Pts',(-6.47468764585225,-0.66166382004421,
2.63046431487488));
#12351=CARTESIAN_POINT('Ctrl Pts',(-6.16628249672348,-0.127049888527898,
2.65276536643547));
#12352=CARTESIAN_POINT('Ctrl Pts',(-6.28109568951485,0.372277207765494,
2.67131565746007));
#12353=CARTESIAN_POINT('Ctrl Pts',(-6.5572455755856,0.646536190026674,2.68613740871844));
#12354=CARTESIAN_POINT('Ctrl Pts',(-6.82386434223888,0.763331776026648,
2.69724384027595));
#12355=CARTESIAN_POINT('Ctrl Pts',(-7.11493971367238,0.774008603859367,
2.70834079855829));
#12356=CARTESIAN_POINT('Ctrl Pts',(-7.38944668657708,0.678048009398333,
2.71942828774665));
#12357=CARTESIAN_POINT('Ctrl Pts',(-7.60966929275022,0.488376278032324,
2.73050641293604));
#12358=CARTESIAN_POINT('Ctrl Pts',(-7.74544261192189,0.231671245772344,
2.74157546675068));
#12359=CARTESIAN_POINT('Ctrl Pts',(-7.77772886818201,-0.0566091099164064,
2.75263518601118));
#12360=CARTESIAN_POINT('Ctrl Pts',(-7.69046381966352,-0.383448777027424,
2.7655283700859));
#12361=CARTESIAN_POINT('Ctrl Pts',(-7.42793832658348,-0.677972215900527,
2.78024752493643));
#12362=CARTESIAN_POINT('Ctrl Pts',(-7.00142534461877,-0.800550675798575,
2.79678644393065));
#12363=CARTESIAN_POINT('Ctrl Pts',(-6.57584982407145,-0.677886291073977,
2.81330669294018));
#12364=CARTESIAN_POINT('Ctrl Pts',(-6.28096997251176,-0.347844732473953,
2.82980813170021));
#12365=CARTESIAN_POINT('Ctrl Pts',(-6.20701576130477,0.087946621438888,
2.84629140165672));
#12366=CARTESIAN_POINT('Ctrl Pts',(-6.37604987195121,0.495869638733109,
2.86275677095718));
#12367=CARTESIAN_POINT('Ctrl Pts',(-6.73581844360051,0.751061859313513,
2.87920481096959));
#12368=CARTESIAN_POINT('Ctrl Pts',(-7.17579711332225,0.775699888633669,
2.89563572893505));
#12369=CARTESIAN_POINT('Ctrl Pts',(-7.56098334322159,0.562728770502053,
2.91205046024346));
#12370=CARTESIAN_POINT('Ctrl Pts',(-7.77381762277454,0.177780339918829,
2.9284483865883));
#12371=CARTESIAN_POINT('Ctrl Pts',(-7.74883414009467,-0.260807751918227,
2.94483239278502));
#12372=CARTESIAN_POINT('Ctrl Pts',(-7.49484470645772,-0.618768936824925,
2.96120009423831));
#12373=CARTESIAN_POINT('Ctrl Pts',(-7.08967346068793,-0.786546626739717,
2.97755335807742));
#12374=CARTESIAN_POINT('Ctrl Pts',(-6.657720721054,-0.713102971741213,2.99389252871196));
#12375=CARTESIAN_POINT('Ctrl Pts',(-6.33131642826648,-0.421337174951404,
3.01021815369535));
#12376=CARTESIAN_POINT('Ctrl Pts',(-6.21026692128662,-0.000967189591566242,
3.02653071397231));
#12377=CARTESIAN_POINT('Ctrl Pts',(-6.33132572760332,0.419054026871033,
3.04283074169105));
#12378=CARTESIAN_POINT('Ctrl Pts',(-6.65705238030844,0.710078042192075,
3.05911874973318));
#12379=CARTESIAN_POINT('Ctrl Pts',(-7.08738278568895,0.783150283438538,
3.07539527341508));
#12380=CARTESIAN_POINT('Ctrl Pts',(-7.49036008893511,0.61618814273907,3.09166084345137));
#12381=CARTESIAN_POINT('Ctrl Pts',(-7.74258151597761,0.260650101302873,
3.10791600264155));
#12382=CARTESIAN_POINT('Ctrl Pts',(-7.76697304166341,-0.174317653031718,
3.12416129945641));
#12383=CARTESIAN_POINT('Ctrl Pts',(-7.5563317668102,-0.555374412970227,
3.14039727791897));
#12384=CARTESIAN_POINT('Ctrl Pts',(-7.17544889508143,-0.765844413327437,
3.15662450083269));
#12385=CARTESIAN_POINT('Ctrl Pts',(-6.74118880081162,-0.74142681352133,
3.17284352210207));
#12386=CARTESIAN_POINT('Ctrl Pts',(-6.38664706125572,-0.489831708198072,
3.18905490924575));
#12387=CARTESIAN_POINT('Ctrl Pts',(-6.22037527072638,-0.0883484616098797,
3.20525922558141));
#12388=CARTESIAN_POINT('Ctrl Pts',(-6.29315956054544,0.339887540079846,
3.22145704360919));
#12389=CARTESIAN_POINT('Ctrl Pts',(-6.58251550195127,0.663644624899192,
3.23764893882998));
#12390=CARTESIAN_POINT('Ctrl Pts',(-6.99963072329188,0.783793247219456,
3.2538354815312));
#12391=CARTESIAN_POINT('Ctrl Pts',(-7.41661272017152,0.663644809896155,
3.27001725696222));
#12392=CARTESIAN_POINT('Ctrl Pts',(-7.70568527679105,0.340149677083231,
3.28619484143681));
#12393=CARTESIAN_POINT('Ctrl Pts',(-7.7783261618395,-0.0874615956887984,
3.30236882102331));
#12394=CARTESIAN_POINT('Ctrl Pts',(-7.61236302022633,-0.488103619326867,
3.31853977629767));
#12395=CARTESIAN_POINT('Ctrl Pts',(-7.25873847420674,-0.739003460387096,
3.33470829571519));
#12396=CARTESIAN_POINT('Ctrl Pts',(-6.82587846889915,-0.763306477612443,
3.35087496493719));
#12397=CARTESIAN_POINT('Ctrl Pts',(-6.44646523023161,-0.55360846219804,
3.36704036914161));
#12398=CARTESIAN_POINT('Ctrl Pts',(-6.23677704618538,-0.174209133649937,
3.38320509172753));
#12399=CARTESIAN_POINT('Ctrl Pts',(-6.26108481548361,0.258592599799861,
3.39936973132143));
#12400=CARTESIAN_POINT('Ctrl Pts',(-6.51192371113038,0.612138413508131,
3.41553483603588));
#12401=CARTESIAN_POINT('Ctrl Pts',(-6.91246725256316,0.778040033227508,
3.43170106480072));
#12402=CARTESIAN_POINT('Ctrl Pts',(-7.33986110031951,0.705423732658014,
3.44786881262982));
#12403=CARTESIAN_POINT('Ctrl Pts',(-7.66330225180869,0.416455198735406,
3.46403905603656));
#12404=CARTESIAN_POINT('Ctrl Pts',(-7.76314448110752,0.0691836941953803,
3.47751601213562));
#12405=CARTESIAN_POINT('Ctrl Pts',(-7.72348592779732,-0.208769115260678,
3.48830037788075));
#12406=CARTESIAN_POINT('Ctrl Pts',(-7.60915687709694,-0.465286651701113,
3.49908593215301));
#12407=CARTESIAN_POINT('Ctrl Pts',(-7.33982769226549,-0.706235104211514,
3.51256903136456));
#12408=CARTESIAN_POINT('Ctrl Pts',(-6.91163155362933,-0.779188237324528,
3.52875357310865));
#12409=CARTESIAN_POINT('Ctrl Pts',(-6.55548444266184,-0.63109352619522,
3.54314470826614));
#12410=CARTESIAN_POINT('Ctrl Pts',(-6.34011871400958,-0.38036708219665,
3.55574171383355));
#12411=CARTESIAN_POINT('Ctrl Pts',(-6.24639647450997,-0.113075731347263,
3.56654128345746));
#12412=CARTESIAN_POINT('Ctrl Pts',(-6.2571004711447,0.170138823557678,3.57734399581171));
#12413=CARTESIAN_POINT('Ctrl Pts',(-6.37034993489611,0.429980603706305,
3.58814957433025));
#12414=CARTESIAN_POINT('Ctrl Pts',(-6.57092700052057,0.630418764957175,
3.59895848058192));
#12415=CARTESIAN_POINT('Ctrl Pts',(-6.830850714758,0.743936015163079,3.60977063520182));
#12416=CARTESIAN_POINT('Ctrl Pts',(-7.11441971427059,0.754517996689564,
3.62058700132255));
#12417=CARTESIAN_POINT('Ctrl Pts',(-7.32278052411025,0.68159756714758,3.62900216988483));
#12418=CARTESIAN_POINT('Ctrl Pts',(-7.50391457198171,0.561381429877749,
3.6374197054472));
#12419=CARTESIAN_POINT('Ctrl Pts',(-7.67348487864857,0.374325256349744,
3.64704230565885));
#12420=CARTESIAN_POINT('Ctrl Pts',(-7.77729848202131,0.0380717430195915,
3.66027880858025));
#12421=CARTESIAN_POINT('Ctrl Pts',(-7.69804120365716,-0.354373328164954,
3.67532745719795));
#12422=CARTESIAN_POINT('Ctrl Pts',(-7.41848398951318,-0.667534119421154,
3.69098736267498));
#12423=CARTESIAN_POINT('Ctrl Pts',(-6.9990632960658,-0.788379913874128,
3.70726054669447));
#12424=CARTESIAN_POINT('Ctrl Pts',(-6.57948025538097,-0.667512143973283,
3.72354511539254));
#12425=CARTESIAN_POINT('Ctrl Pts',(-6.28822210540625,-0.341703386586052,
3.73984162248617));
#12426=CARTESIAN_POINT('Ctrl Pts',(-6.214947252681,0.0895247616185924,3.75615047657178));
#12427=CARTESIAN_POINT('Ctrl Pts',(-6.38236889523311,0.493801790031738,
3.77247232162259));
#12428=CARTESIAN_POINT('Ctrl Pts',(-6.73967995056519,0.747643053294839,
3.78880728997579));
#12429=CARTESIAN_POINT('Ctrl Pts',(-7.12863355815078,0.768970568205483,
3.80334000325068));
#12430=CARTESIAN_POINT('Ctrl Pts',(-7.43455531549802,0.635168646195069,
3.81606611806074));
#12431=CARTESIAN_POINT('Ctrl Pts',(-7.6371093846873,0.432883606871512,3.8269804250519));
#12432=CARTESIAN_POINT('Ctrl Pts',(-7.75160187649833,0.170239682165284,
3.8379015715229));
#12433=CARTESIAN_POINT('Ctrl Pts',(-7.76244105669299,-0.116247652674151,
3.84882949139145));
#12434=CARTESIAN_POINT('Ctrl Pts',(-7.66763793861865,-0.386911128974891,
3.85976441318346));
#12435=CARTESIAN_POINT('Ctrl Pts',(-7.48047767628426,-0.604726336185073,
3.87070649501486));
#12436=CARTESIAN_POINT('Ctrl Pts',(-7.22657273961852,-0.738431388646221,
3.88165581413315));
#12437=CARTESIAN_POINT('Ctrl Pts',(-6.84559484715752,-0.782659505496549,
3.89626492121388));
#12438=CARTESIAN_POINT('Ctrl Pts',(-6.39035895969544,-0.564314377486963,
3.91454454394013));
#12439=CARTESIAN_POINT('Ctrl Pts',(-6.16773943366211,0.00142552218543602,
3.93651217130362));
#12440=CARTESIAN_POINT('Ctrl Pts',(-6.39017049813292,0.567679522925422,
3.95851150179096));
#12441=CARTESIAN_POINT('Ctrl Pts',(-6.93898016017053,0.83229149877013,3.98054457232659));
#12442=CARTESIAN_POINT('Ctrl Pts',(-7.52223705917294,0.652480441661669,
4.0026118930303));
#12443=CARTESIAN_POINT('Ctrl Pts',(-7.82804385744497,0.123409451029175,
4.02471464764302));
#12444=CARTESIAN_POINT('Ctrl Pts',(-7.69193113695034,-0.473949690379908,
4.04685362373763));
#12445=CARTESIAN_POINT('Ctrl Pts',(-7.24181863438223,-0.780329262527218,
4.06656588170735));
#12446=CARTESIAN_POINT('Ctrl Pts',(-6.7820134805878,-0.767442446346911,
4.08383853386223));
#12447=CARTESIAN_POINT('Ctrl Pts',(-6.44086041985743,-0.571004816225905,
4.09866082654509));
#12448=CARTESIAN_POINT('Ctrl Pts',(-6.2349792076924,-0.234034685896682,
4.11350056349035));
#12449=CARTESIAN_POINT('Ctrl Pts',(-6.21504713433741,0.160446370067885,
4.12835806169351));
#12450=CARTESIAN_POINT('Ctrl Pts',(-6.3868236701026,0.51690216155789,4.14323345115286));
#12451=CARTESIAN_POINT('Ctrl Pts',(-6.68160097485276,0.728706442019366,
4.15688557825564));
#12452=CARTESIAN_POINT('Ctrl Pts',(-7.0019056807236,0.789135115020865,4.16931021399055));
#12453=CARTESIAN_POINT('Ctrl Pts',(-7.29042452641039,0.734688640425214,
4.18050272820112));
#12454=CARTESIAN_POINT('Ctrl Pts',(-7.53916074485403,0.578311269612235,
4.19170571187556));
#12455=CARTESIAN_POINT('Ctrl Pts',(-7.71409171667038,0.341590655634556,
4.20291927766093));
#12456=CARTESIAN_POINT('Ctrl Pts',(-7.7898177049696,0.0574856270825079,
4.21414344977244));
#12457=CARTESIAN_POINT('Ctrl Pts',(-7.74706612373166,-0.333862955380633,
4.22912337531477));
#12458=CARTESIAN_POINT('Ctrl Pts',(-7.48937849541761,-0.657211178204218,
4.24412476954085));
#12459=CARTESIAN_POINT('Ctrl Pts',(-7.11628554615372,-0.786433878154665,
4.25914816467973));
#12460=CARTESIAN_POINT('Ctrl Pts',(-6.82103578880878,-0.77581930313266,
4.2704267350549));
#12461=CARTESIAN_POINT('Ctrl Pts',(-6.5494657022935,-0.657201742063754,
4.28171637563045));
#12462=CARTESIAN_POINT('Ctrl Pts',(-6.33982460180875,-0.447724590754319,
4.29301720482683));
#12463=CARTESIAN_POINT('Ctrl Pts',(-6.2212038304369,-0.175704823349057,
4.30432922595009));
#12464=CARTESIAN_POINT('Ctrl Pts',(-6.20996096390589,0.12113566135513,4.31565255452681));
#12465=CARTESIAN_POINT('Ctrl Pts',(-6.3082813903755,0.401676910179385,4.32698721417064));
#12466=CARTESIAN_POINT('Ctrl Pts',(-6.53453931041383,0.665155379172314,
4.34022426133603));
#12467=CARTESIAN_POINT('Ctrl Pts',(-6.90934792817869,0.821130796703102,
4.3553714888365));
#12468=CARTESIAN_POINT('Ctrl Pts',(-7.36074527364388,0.744316254597853,
4.37243815749654));
#12469=CARTESIAN_POINT('Ctrl Pts',(-7.7024754750817,0.43907929924283,4.38953088858621));
#12470=CARTESIAN_POINT('Ctrl Pts',(-7.82969309329709,-0.00204137070426244,
4.40664990380937));
#12471=CARTESIAN_POINT('Ctrl Pts',(-7.70250067292396,-0.443824957085235,
4.42379531432277));
#12472=CARTESIAN_POINT('Ctrl Pts',(-7.3592455074783,-0.750732264321921,
4.44096726291832));
#12473=CARTESIAN_POINT('Ctrl Pts',(-6.90461076111005,-0.828077026739987,
4.45816585671055));
#12474=CARTESIAN_POINT('Ctrl Pts',(-6.47785145640082,-0.651418695241634,
4.47539120143168));
#12475=CARTESIAN_POINT('Ctrl Pts',(-6.21007591581231,-0.274199129165646,
4.49264338319947));
#12476=CARTESIAN_POINT('Ctrl Pts',(-6.18399470172574,0.188387346819458,
4.50992248166671));
#12477=CARTESIAN_POINT('Ctrl Pts',(-6.40837539543801,0.594574778942697,
4.52722855314471));
#12478=CARTESIAN_POINT('Ctrl Pts',(-6.81509167143493,0.819485331368328,
4.54456166410994));
#12479=CARTESIAN_POINT('Ctrl Pts',(-7.27987319414489,0.793471678330472,
4.56192181882538));
#12480=CARTESIAN_POINT('Ctrl Pts',(-7.66011479470359,0.523796174615442,
4.57930912132998));
#12481=CARTESIAN_POINT('Ctrl Pts',(-7.83898719320449,0.0923657793623214,
4.59672341312303));
#12482=CARTESIAN_POINT('Ctrl Pts',(-7.77359845357327,-0.29173800569068,
4.61125815306387));
#12483=CARTESIAN_POINT('Ctrl Pts',(-7.60486413396222,-0.543478230712311,
4.62289900894297));
#12484=CARTESIAN_POINT('Ctrl Pts',(-7.37344723337822,-0.739509772796316,
4.63454888242984));
#12485=CARTESIAN_POINT('Ctrl Pts',(-6.99796916640192,-0.847988290174798,
4.64912877493909));
#12486=CARTESIAN_POINT('Ctrl Pts',(-6.54638127238998,-0.717940114779771,
4.6666513290107));
#12487=CARTESIAN_POINT('Ctrl Pts',(-6.232781786496,-0.367178113186201,4.68420096407712));
#12488=CARTESIAN_POINT('Ctrl Pts',(-6.15372371672015,0.0974436948677159,
4.70177742940139));
#12489=CARTESIAN_POINT('Ctrl Pts',(-6.33426751835694,0.533542705055676,
4.71938074720947));
#12490=CARTESIAN_POINT('Ctrl Pts',(-6.7197391499259,0.807173042125499,4.73701077817937));
#12491=CARTESIAN_POINT('Ctrl Pts',(-7.19242759577209,0.833802363418686,
4.75466748667689));
#12492=CARTESIAN_POINT('Ctrl Pts',(-7.60745560394516,0.60453864229177,4.77235067103721));
#12493=CARTESIAN_POINT('Ctrl Pts',(-7.83725063197469,0.188941390247915,
4.79006042872509));
#12494=CARTESIAN_POINT('Ctrl Pts',(-7.8106711862218,-0.285829700854973,
4.80779618745207));
#12495=CARTESIAN_POINT('Ctrl Pts',(-7.53521563022957,-0.674475138957433,
4.82555885140828));
#12496=CARTESIAN_POINT('Ctrl Pts',(-7.09452497559831,-0.856799563884475,
4.84334606079258));
#12497=CARTESIAN_POINT('Ctrl Pts',(-6.62369779984497,-0.777148624143293,
4.86115986092763));
#12498=CARTESIAN_POINT('Ctrl Pts',(-6.26696887582568,-0.458201653067476,
4.87899721597154));
#12499=CARTESIAN_POINT('Ctrl Pts',(-6.17856731994658,-0.151930989278767,
4.89090963520109));
#12500=CARTESIAN_POINT('Ctrl Pts',(-6.17854660968293,0.00205226831345774,
4.89686544420304));
#12501=CARTESIAN_POINT('Ctrl Pts',(-6.15532181468697,0.00138488703415226,
1.01435007802725));
#12502=CARTESIAN_POINT('Ctrl Pts',(-6.1553431152372,0.159757645663868,1.02047566534903));
#12503=CARTESIAN_POINT('Ctrl Pts',(-6.24623111421967,0.475075705756006,
1.03273758175489));
#12504=CARTESIAN_POINT('Ctrl Pts',(-6.61422672853683,0.80433161688607,1.05114350930259));
#12505=CARTESIAN_POINT('Ctrl Pts',(-7.10116639540294,0.886859556533852,
1.06956675049812));
#12506=CARTESIAN_POINT('Ctrl Pts',(-7.55806039306351,0.698002185192178,
1.08800459577221));
#12507=CARTESIAN_POINT('Ctrl Pts',(-7.8443721167838,0.294291635454448,1.1064570708697));
#12508=CARTESIAN_POINT('Ctrl Pts',(-7.87219577959167,-0.200096078911815,
1.12492425022168));
#12509=CARTESIAN_POINT('Ctrl Pts',(-7.63250722014404,-0.633915270826186,
1.14340533646129));
#12510=CARTESIAN_POINT('Ctrl Pts',(-7.19844236190399,-0.87385140291206,
1.16189996598086));
#12511=CARTESIAN_POINT('Ctrl Pts',(-6.70297864922338,-0.846086645447464,
1.1804074750247));
#12512=CARTESIAN_POINT('Ctrl Pts',(-6.2978047958826,-0.558728259760231,
1.19892754958468));
#12513=CARTESIAN_POINT('Ctrl Pts',(-6.139538539105,-0.176162993711043,1.2143705962764));
#12514=CARTESIAN_POINT('Ctrl Pts',(-6.14903967530696,0.145501856680318,
1.22673123417169));
#12515=CARTESIAN_POINT('Ctrl Pts',(-6.24632555571259,0.452346696169204,
1.239095571006));
#12516=CARTESIAN_POINT('Ctrl Pts',(-6.52234008288225,0.761589519917251,
1.25455717363935));
#12517=CARTESIAN_POINT('Ctrl Pts',(-7.00080290977026,0.899413229449575,
1.27312169979619));
#12518=CARTESIAN_POINT('Ctrl Pts',(-7.47936561468606,0.761578690439182,
1.29169587691259));
#12519=CARTESIAN_POINT('Ctrl Pts',(-7.81146685686393,0.390026773641098,
1.31027931928451));
#12520=CARTESIAN_POINT('Ctrl Pts',(-7.89499560809641,-0.101473505781537,
1.3288713963235));
#12521=CARTESIAN_POINT('Ctrl Pts',(-7.70415448553098,-0.562288126274461,
1.34747158083016));
#12522=CARTESIAN_POINT('Ctrl Pts',(-7.29722514506761,-0.851048902454855,
1.3660792909068));
#12523=CARTESIAN_POINT('Ctrl Pts',(-6.79885441200529,-0.879060781972192,
1.38469396999124));
#12524=CARTESIAN_POINT('Ctrl Pts',(-6.36181870759125,-0.63754524480614,
1.40331504129361));
#12525=CARTESIAN_POINT('Ctrl Pts',(-6.12019073027554,-0.200394147677602,
1.42194193808049));
#12526=CARTESIAN_POINT('Ctrl Pts',(-6.14818632446221,0.298444301700259,
1.4405740774677));
#12527=CARTESIAN_POINT('Ctrl Pts',(-6.43736173956987,0.706031374616256,
1.45921088701331));
#12528=CARTESIAN_POINT('Ctrl Pts',(-6.89916431053514,0.897327322215646,
1.4778517860215));
#12529=CARTESIAN_POINT('Ctrl Pts',(-7.39204751091533,0.813605469747302,
1.49649618519644));
#12530=CARTESIAN_POINT('Ctrl Pts',(-7.76489965161589,0.480398984552206,
1.51514351443042));
#12531=CARTESIAN_POINT('Ctrl Pts',(-7.90332809212511,-8.96281492521594E-5,
1.53379315987099));
#12532=CARTESIAN_POINT('Ctrl Pts',(-7.7649060157838,-0.480792699234354,
1.55244459112492));
#12533=CARTESIAN_POINT('Ctrl Pts',(-7.45403998538145,-0.75829949879398,
1.56798834125249));
#12534=CARTESIAN_POINT('Ctrl Pts',(-7.14544718809111,-0.856141214202644,
1.58042376628376));
#12535=CARTESIAN_POINT('Ctrl Pts',(-6.82180196362564,-0.865733441257941,
1.592859283437));
#12536=CARTESIAN_POINT('Ctrl Pts',(-6.45398629112311,-0.713440752735991,
1.60771267399531));
#12537=CARTESIAN_POINT('Ctrl Pts',(-6.17673186358275,-0.347059455508924,
1.62498362624803));
#12538=CARTESIAN_POINT('Ctrl Pts',(-6.11099778616178,0.0887865953086014,
1.64156282477639));
#12539=CARTESIAN_POINT('Ctrl Pts',(-6.26177741085195,0.503103111464865,
1.6581407399915));
#12540=CARTESIAN_POINT('Ctrl Pts',(-6.5923194610229,0.794739465687361,1.67471694279706));
#12541=CARTESIAN_POINT('Ctrl Pts',(-7.02193769700808,0.892823305180966,
1.69129102758754));
#12542=CARTESIAN_POINT('Ctrl Pts',(-7.44632452845763,0.773409502201043,
1.70786259019089));
#12543=CARTESIAN_POINT('Ctrl Pts',(-7.76130934158841,0.46580285735598,1.72443120336651));
#12544=CARTESIAN_POINT('Ctrl Pts',(-7.90651951677609,-0.00196807962334312,
1.74283704477602));
#12545=CARTESIAN_POINT('Ctrl Pts',(-7.75330353635983,-0.531346850232141,
1.76307810860955));
#12546=CARTESIAN_POINT('Ctrl Pts',(-7.26449796556357,-0.882702447669824,
1.78515164667195));
#12547=CARTESIAN_POINT('Ctrl Pts',(-6.71436229145052,-0.859335279308994,
1.80537779316638));
#12548=CARTESIAN_POINT('Ctrl Pts',(-6.3176646664297,-0.573013323811329,
1.82375837638183));
#12549=CARTESIAN_POINT('Ctrl Pts',(-6.12680833020744,-0.177218873527421,
1.84029511474842));
#12550=CARTESIAN_POINT('Ctrl Pts',(-6.14875890700447,0.261990487464417,
1.85682569031829));
#12551=CARTESIAN_POINT('Ctrl Pts',(-6.37791553494525,0.636870862801446,
1.87334973144588));
#12552=CARTESIAN_POINT('Ctrl Pts',(-6.7582629833497,0.856443868873814,1.8898667925222));
#12553=CARTESIAN_POINT('Ctrl Pts',(-7.19729006439147,0.867492922871737,
1.90637662966974));
#12554=CARTESIAN_POINT('Ctrl Pts',(-7.52245896265695,0.700396003581133,
1.92012822956414));
#12555=CARTESIAN_POINT('Ctrl Pts',(-7.71126282344545,0.485974231171035,
1.93112537636886));
#12556=CARTESIAN_POINT('Ctrl Pts',(-7.84183705801084,0.231956797192165,
1.94211976155069));
#12557=CARTESIAN_POINT('Ctrl Pts',(-7.87828239403315,-0.131509317473049,
1.95585786032622));
#12558=CARTESIAN_POINT('Ctrl Pts',(-7.70820816241811,-0.535261941489649,
1.97233415651205));
#12559=CARTESIAN_POINT('Ctrl Pts',(-7.36572329095194,-0.80840715001223,
1.98880189639337));
#12560=CARTESIAN_POINT('Ctrl Pts',(-6.97067541231049,-0.877668187533008,
2.00388811678008));
#12561=CARTESIAN_POINT('Ctrl Pts',(-6.62339026681109,-0.78435311697415,
2.01759537265686));
#12562=CARTESIAN_POINT('Ctrl Pts',(-6.3630812755978,-0.592396239794856,
2.02992631914616));
#12563=CARTESIAN_POINT('Ctrl Pts',(-6.19117506852127,-0.318573480034593,
2.04225125653785));
#12564=CARTESIAN_POINT('Ctrl Pts',(-6.13101025620552,-0.0010421798929461,
2.05457019344336));
#12565=CARTESIAN_POINT('Ctrl Pts',(-6.19117175900474,0.316205694335182,
2.06688287651045));
#12566=CARTESIAN_POINT('Ctrl Pts',(-6.36285264509343,0.589792470866144,
2.07918920353492));
#12567=CARTESIAN_POINT('Ctrl Pts',(-6.62249464601974,0.780782662724837,
2.09148902616807));
#12568=CARTESIAN_POINT('Ctrl Pts',(-7.0378498001605,0.89353864001136,2.10787980243138));
#12569=CARTESIAN_POINT('Ctrl Pts',(-7.57827502836269,0.727484904857922,
2.12835184441199));
#12570=CARTESIAN_POINT('Ctrl Pts',(-7.91766293688888,0.139356339769869,
2.15288956866496));
#12571=CARTESIAN_POINT('Ctrl Pts',(-7.76659689250598,-0.521123950569987,
2.17739794495675));
#12572=CARTESIAN_POINT('Ctrl Pts',(-7.20729504630159,-0.902360411029734,
2.20187569995981));
#12573=CARTESIAN_POINT('Ctrl Pts',(-6.53885375332028,-0.801399036365866,
2.2263218674333));
#12574=CARTESIAN_POINT('Ctrl Pts',(-6.11808523348063,-0.273493855561213,
2.25073537703529));
#12575=CARTESIAN_POINT('Ctrl Pts',(-6.16864061548512,0.398778645678198,
2.27511524207653));
#12576=CARTESIAN_POINT('Ctrl Pts',(-6.66226090036659,0.856536394347886,
2.29946047535543));
#12577=CARTESIAN_POINT('Ctrl Pts',(-7.33447899690987,0.856349278793802,
2.32377013175939));
#12578=CARTESIAN_POINT('Ctrl Pts',(-7.82637817814363,0.399669335099744,
2.34804328860591));
#12579=CARTESIAN_POINT('Ctrl Pts',(-7.8762624403739,-0.268644644505232,
2.3722790575478));
#12580=CARTESIAN_POINT('Ctrl Pts',(-7.45891773050366,-0.791653462716088,
2.39647657914323));
#12581=CARTESIAN_POINT('Ctrl Pts',(-6.79831471817344,-0.891013892478177,
2.42063502780583));
#12582=CARTESIAN_POINT('Ctrl Pts',(-6.24739027927042,-0.515144657685069,
2.44475360957481));
#12583=CARTESIAN_POINT('Ctrl Pts',(-6.09944401021374,0.134016413694163,
2.46883156460017));
#12584=CARTESIAN_POINT('Ctrl Pts',(-6.43196540399374,0.709519549341717,
2.49286816857682));
#12585=CARTESIAN_POINT('Ctrl Pts',(-7.06605101482765,0.904879456246692,
2.51686272802793));
#12586=CARTESIAN_POINT('Ctrl Pts',(-7.6626855728488,0.617300900309224,2.54081459614203));
#12587=CARTESIAN_POINT('Ctrl Pts',(-7.90400060789426,0.00181430507667405,
2.56472313989482));
#12588=CARTESIAN_POINT('Ctrl Pts',(-7.66272120125994,-0.612424319707219,
2.58858781519659));
#12589=CARTESIAN_POINT('Ctrl Pts',(-7.06913692438929,-0.897923665578739,
2.61240800689291));
#12590=CARTESIAN_POINT('Ctrl Pts',(-6.44110784712269,-0.704106841661814,
2.63618339293661));
#12591=CARTESIAN_POINT('Ctrl Pts',(-6.11300163800619,-0.13530675007174,
2.6599131277551));
#12592=CARTESIAN_POINT('Ctrl Pts',(-6.23516444880693,0.395865212665747,
2.67965031459637));
#12593=CARTESIAN_POINT('Ctrl Pts',(-6.52887561201059,0.687563852182344,
2.69541600209137));
#12594=CARTESIAN_POINT('Ctrl Pts',(-6.81242451351045,0.811765155919268,
2.70722885200896));
#12595=CARTESIAN_POINT('Ctrl Pts',(-7.12193899701994,0.823119375286228,
2.71902998121532));
#12596=CARTESIAN_POINT('Ctrl Pts',(-7.41379212450475,0.721083917159786,
2.73081943099457));
#12597=CARTESIAN_POINT('Ctrl Pts',(-7.64789851807236,0.519457544257522,
2.74259717622193));
#12598=CARTESIAN_POINT('Ctrl Pts',(-7.79219812426804,0.246613467879735,
2.75436301193177));
#12599=CARTESIAN_POINT('Ctrl Pts',(-7.82650908620457,-0.0597313562161861,
2.7661172444166));
#12600=CARTESIAN_POINT('Ctrl Pts',(-7.73378757716163,-0.406973488614899,
2.77981611351335));
#12601=CARTESIAN_POINT('Ctrl Pts',(-7.45492482469592,-0.71980366041697,
2.7954531697841));
#12602=CARTESIAN_POINT('Ctrl Pts',(-7.00202657290324,-0.849945537810255,
2.81301855620783));
#12603=CARTESIAN_POINT('Ctrl Pts',(-6.55031472914827,-0.719724882478119,
2.83055666346136));
#12604=CARTESIAN_POINT('Ctrl Pts',(-6.23746400207544,-0.36953503313781,
2.84806791497705));
#12605=CARTESIAN_POINT('Ctrl Pts',(-6.15906083953478,0.0926443368691964,
2.86555208259416));
#12606=CARTESIAN_POINT('Ctrl Pts',(-6.33827503896183,0.525051519501817,
2.88300927653526));
#12607=CARTESIAN_POINT('Ctrl Pts',(-6.71948296038623,0.795408929008851,
2.9004393700713));
#12608=CARTESIAN_POINT('Ctrl Pts',(-7.18541682404627,0.821461485746422,
2.91784256578514));
#12609=CARTESIAN_POINT('Ctrl Pts',(-7.59308397004501,0.596020867715862,
2.93521846564008));
#12610=CARTESIAN_POINT('Ctrl Pts',(-7.81818529244133,0.188794732061472,
2.95256800644698));
#12611=CARTESIAN_POINT('Ctrl Pts',(-7.7917393257621,-0.274841348485349,
2.96988919463305));
#12612=CARTESIAN_POINT('Ctrl Pts',(-7.52336307186317,-0.652997969583897,
2.98718447937879));
#12613=CARTESIAN_POINT('Ctrl Pts',(-7.09557333299563,-0.830093838469998,
3.00445276553991));
#12614=CARTESIAN_POINT('Ctrl Pts',(-6.63984770037723,-0.752562258100537,
3.02169424976486));
#12615=CARTESIAN_POINT('Ctrl Pts',(-6.29575429265797,-0.444921405411109,
3.03890898207291));
#12616=CARTESIAN_POINT('Ctrl Pts',(-6.16827535941431,-0.0020478494357645,
3.05609707435848));
#12617=CARTESIAN_POINT('Ctrl Pts',(-6.29576084516153,0.440087461163198,
3.07325862942099));
#12618=CARTESIAN_POINT('Ctrl Pts',(-6.63840792454696,0.746158494232759,
3.09039376920604));
#12619=CARTESIAN_POINT('Ctrl Pts',(-7.09068019304077,0.822901273377244,
3.10750262488744));
#12620=CARTESIAN_POINT('Ctrl Pts',(-7.51381249206245,0.647527693807565,
3.12458534015527));
#12621=CARTESIAN_POINT('Ctrl Pts',(-7.77838184349055,0.274483967111054,
3.1416420706223));
#12622=CARTESIAN_POINT('Ctrl Pts',(-7.80388976455076,-0.181448994759944,
3.15867298547141));
#12623=CARTESIAN_POINT('Ctrl Pts',(-7.5832500525651,-0.580467956848055,
3.17567826210021));
#12624=CARTESIAN_POINT('Ctrl Pts',(-7.18473556223459,-0.800610040459843,
3.19265809517254));
#12625=CARTESIAN_POINT('Ctrl Pts',(-6.73085657140814,-0.775025767238161,
3.20961268663487));
#12626=CARTESIAN_POINT('Ctrl Pts',(-6.36070451906988,-0.512273567169555,
3.22654225372828));
#12627=CARTESIAN_POINT('Ctrl Pts',(-6.18733396966188,-0.0934765731086235,
3.24344702281474));
#12628=CARTESIAN_POINT('Ctrl Pts',(-6.26323916414107,0.352718866884148,
3.26032723384026));
#12629=CARTESIAN_POINT('Ctrl Pts',(-6.5644653146297,0.689654189913989,3.27718313896965));
#12630=CARTESIAN_POINT('Ctrl Pts',(-6.99816156269536,0.814506053793651,
3.29401499779763));
#12631=CARTESIAN_POINT('Ctrl Pts',(-7.43119591985385,0.689658200052887,
3.31082308735104));
#12632=CARTESIAN_POINT('Ctrl Pts',(-7.73101487965898,0.354028369562565,
3.32760769072432));
#12633=CARTESIAN_POINT('Ctrl Pts',(-7.80621008929764,-0.0890580187097431,
3.34436910576017));
#12634=CARTESIAN_POINT('Ctrl Pts',(-7.63437921518094,-0.503670252109045,
3.3611076385834));
#12635=CARTESIAN_POINT('Ctrl Pts',(-7.26879300011845,-0.762964363645185,
3.37782360837663));
#12636=CARTESIAN_POINT('Ctrl Pts',(-6.82188403144782,-0.787979502772466,
3.39451734656986));
#12637=CARTESIAN_POINT('Ctrl Pts',(-6.43068068140195,-0.571676584050765,
3.41118918856227));
#12638=CARTESIAN_POINT('Ctrl Pts',(-6.21479487163316,-0.180901065491681,
3.42783949414826));
#12639=CARTESIAN_POINT('Ctrl Pts',(-6.23987688745805,0.264266034793347,
3.44446861244254));
#12640=CARTESIAN_POINT('Ctrl Pts',(-6.49762030296562,0.627403516828641,
3.46107694553375));
#12641=CARTESIAN_POINT('Ctrl Pts',(-6.90858155892206,0.79753201259649,3.47766481821013));
#12642=CARTESIAN_POINT('Ctrl Pts',(-7.34647065959468,0.723048174829234,
3.49423276489497));
#12643=CARTESIAN_POINT('Ctrl Pts',(-7.67737022510294,0.427306551784298,
3.51078089929711));
#12644=CARTESIAN_POINT('Ctrl Pts',(-7.77933122717147,0.0724197403299812,
3.52455543522332));
#12645=CARTESIAN_POINT('Ctrl Pts',(-7.73883473089208,-0.211307153844965,
3.53556486182041));
#12646=CARTESIAN_POINT('Ctrl Pts',(-7.62219195347972,-0.472977173161771,
3.54656812666788));
#12647=CARTESIAN_POINT('Ctrl Pts',(-7.34766442127358,-0.718477552599507,
3.56031169704533));
#12648=CARTESIAN_POINT('Ctrl Pts',(-6.91186389572488,-0.792629818951791,
3.57678586132189));
#12649=CARTESIAN_POINT('Ctrl Pts',(-6.54994772408427,-0.642052793745427,
3.59141379637521));
#12650=CARTESIAN_POINT('Ctrl Pts',(-6.33135654406045,-0.387527817989315,
3.60420144661415));
#12651=CARTESIAN_POINT('Ctrl Pts',(-6.23633570855798,-0.116439386124594,
3.61515526155727));
#12652=CARTESIAN_POINT('Ctrl Pts',(-6.24720382915164,0.170515824271984,
3.62610159770129));
#12653=CARTESIAN_POINT('Ctrl Pts',(-6.36187322079165,0.433535026443583,
3.63704090051234));
#12654=CARTESIAN_POINT('Ctrl Pts',(-6.56473431971144,0.636227626371285,
3.64797311424009));
#12655=CARTESIAN_POINT('Ctrl Pts',(-6.82736797498893,0.750897209952491,
3.658898542734));
#12656=CARTESIAN_POINT('Ctrl Pts',(-7.11359555037847,0.761558159597187,
3.66981678486612));
#12657=CARTESIAN_POINT('Ctrl Pts',(-7.32371319540262,0.688003016744239,
3.67830393871623));
#12658=CARTESIAN_POINT('Ctrl Pts',(-7.50625823729936,0.566851651520274,
3.68678751070037));
#12659=CARTESIAN_POINT('Ctrl Pts',(-7.67702206646534,0.378444857690304,
3.69647907721837));
#12660=CARTESIAN_POINT('Ctrl Pts',(-7.78141257136081,0.0401475505155527,
3.70979636942345));
#12661=CARTESIAN_POINT('Ctrl Pts',(-7.70171508493293,-0.354162708398042,
3.72491902485287));
#12662=CARTESIAN_POINT('Ctrl Pts',(-7.42114612466325,-0.668341455127249,
3.74063460686844));
#12663=CARTESIAN_POINT('Ctrl Pts',(-7.00088080163629,-0.789344259007442,
3.75694185015021));
#12664=CARTESIAN_POINT('Ctrl Pts',(-6.58110712328952,-0.668334279667831,
3.77323691251503));
#12665=CARTESIAN_POINT('Ctrl Pts',(-6.29018412194349,-0.34277049623807,
3.78952031471304));
#12666=CARTESIAN_POINT('Ctrl Pts',(-6.21717139609482,0.0874524632090739,
3.80579265961626));
#12667=CARTESIAN_POINT('Ctrl Pts',(-6.38403928177642,0.490161525526526,
3.82205440992407));
#12668=CARTESIAN_POINT('Ctrl Pts',(-6.73954376788978,0.742605706624229,
3.83830635307579));
#12669=CARTESIAN_POINT('Ctrl Pts',(-7.1259124951814,0.763713676639482,3.85274389917685));
#12670=CARTESIAN_POINT('Ctrl Pts',(-7.42942016411094,0.630936102189617,
3.86537059518623));
#12671=CARTESIAN_POINT('Ctrl Pts',(-7.6301784569546,0.430405395217166,3.87618990189906));
#12672=CARTESIAN_POINT('Ctrl Pts',(-7.74353726685436,0.170304121516873,
3.88700551322282));
#12673=CARTESIAN_POINT('Ctrl Pts',(-7.75423281912403,-0.113134514061421,
3.89781770500068));
#12674=CARTESIAN_POINT('Ctrl Pts',(-7.66050792598422,-0.380656665238867,
3.90862661199449));
#12675=CARTESIAN_POINT('Ctrl Pts',(-7.47566669878727,-0.595729520002875,
3.91943237649964));
#12676=CARTESIAN_POINT('Ctrl Pts',(-7.22516692240344,-0.727621081205731,
3.93023521909756));
#12677=CARTESIAN_POINT('Ctrl Pts',(-6.84964587248811,-0.771177648449039,
3.94463520824916));
#12678=CARTESIAN_POINT('Ctrl Pts',(-6.40163159698102,-0.556119063029255,
3.96262903315017));
#12679=CARTESIAN_POINT('Ctrl Pts',(-6.18311346213355,-0.000224236590168895,
3.98421206227288));
#12680=CARTESIAN_POINT('Ctrl Pts',(-6.40142810194215,0.555005154061987,
4.00578771530793));
#12681=CARTESIAN_POINT('Ctrl Pts',(-6.93874203129211,0.813853076380022,
4.02735679834234));
#12682=CARTESIAN_POINT('Ctrl Pts',(-7.50861106416408,0.637962848998229,
4.04892096810037));
#12683=CARTESIAN_POINT('Ctrl Pts',(-7.80673620650473,0.121794509865376,
4.07048149068405));
#12684=CARTESIAN_POINT('Ctrl Pts',(-7.67400892248061,-0.459829671966149,
4.0920398259536));
#12685=CARTESIAN_POINT('Ctrl Pts',(-7.23638059365412,-0.75751561964237,
4.11120202311155));
#12686=CARTESIAN_POINT('Ctrl Pts',(-6.79005425730626,-0.744940744569275,
4.1279693946883));
#12687=CARTESIAN_POINT('Ctrl Pts',(-6.45928263693368,-0.554426517452247,
4.14234208150331));
#12688=CARTESIAN_POINT('Ctrl Pts',(-6.25991541608282,-0.228019663351229,
4.15671586125759));
#12689=CARTESIAN_POINT('Ctrl Pts',(-6.24068116030339,0.15365327946892,4.1710910801691));
#12690=CARTESIAN_POINT('Ctrl Pts',(-6.40674558298073,0.498142296774453,
4.1854682482322));
#12691=CARTESIAN_POINT('Ctrl Pts',(-6.69137279180131,0.702599429114232,
4.19864939667764));
#12692=CARTESIAN_POINT('Ctrl Pts',(-7.00034153191099,0.760867123384676,
4.21063430004806));
#12693=CARTESIAN_POINT('Ctrl Pts',(-7.27843068823313,0.70836902278032,4.22142238458483));
#12694=CARTESIAN_POINT('Ctrl Pts',(-7.5179857131659,0.557741775949331,4.23221238061628));
#12695=CARTESIAN_POINT('Ctrl Pts',(-7.68632465558915,0.329907804903081,
4.24300440013838));
#12696=CARTESIAN_POINT('Ctrl Pts',(-7.75913469605848,0.0566828026146494,
4.25379865262834));
#12697=CARTESIAN_POINT('Ctrl Pts',(-7.7180202023265,-0.319402775086334,
4.26819421301669));
#12698=CARTESIAN_POINT('Ctrl Pts',(-7.47057957124159,-0.629743130547593,
4.28259470202932));
#12699=CARTESIAN_POINT('Ctrl Pts',(-7.11280162175997,-0.753630952420848,
4.29700123189475));
#12700=CARTESIAN_POINT('Ctrl Pts',(-6.82986918527034,-0.743445233993496,
4.30780913559938));
#12701=CARTESIAN_POINT('Ctrl Pts',(-6.56981457045782,-0.629837115749421,
4.31862032283963));
#12702=CARTESIAN_POINT('Ctrl Pts',(-6.36920262800273,-0.429359709312094,
4.32943489251995));
#12703=CARTESIAN_POINT('Ctrl Pts',(-6.25577547078144,-0.169206543388766,
4.34025305726424));
#12704=CARTESIAN_POINT('Ctrl Pts',(-6.24504644209274,0.114494238429322,
4.35107497032088));
#12705=CARTESIAN_POINT('Ctrl Pts',(-6.33896947900305,0.38243886083468,4.36190076276199));
#12706=CARTESIAN_POINT('Ctrl Pts',(-6.55495387030909,0.633924630661768,
4.37453573308082));
#12707=CARTESIAN_POINT('Ctrl Pts',(-6.9124614167636,0.782648524492007,4.38898251478319));
#12708=CARTESIAN_POINT('Ctrl Pts',(-7.34259808028965,0.709396411557978,
4.40524507600026));
#12709=CARTESIAN_POINT('Ctrl Pts',(-7.66792322353676,0.418743989320809,
4.42151836634654));
#12710=CARTESIAN_POINT('Ctrl Pts',(-7.78889500630819,-0.000902978993542901,
4.43780279177667));
#12711=CARTESIAN_POINT('Ctrl Pts',(-7.66795110493541,-0.420807930740282,
4.45409892771709));
#12712=CARTESIAN_POINT('Ctrl Pts',(-7.34191240663444,-0.712259181511612,
4.47040727724938));
#12713=CARTESIAN_POINT('Ctrl Pts',(-6.91044557617938,-0.785616858356274,
4.4867283632995));
#12714=CARTESIAN_POINT('Ctrl Pts',(-6.50575685387359,-0.618047933668166,
4.50306269522463));
#12715=CARTESIAN_POINT('Ctrl Pts',(-6.25203399164393,-0.260552904403482,
4.51941078451858));
#12716=CARTESIAN_POINT('Ctrl Pts',(-6.22737477948063,0.17751833719177,4.53577312557919));
#12717=CARTESIAN_POINT('Ctrl Pts',(-6.43975685988429,0.561906946644777,
4.5521502223111));
#12718=CARTESIAN_POINT('Ctrl Pts',(-6.82444025681707,0.774592630399746,
4.56854254120903));
#12719=CARTESIAN_POINT('Ctrl Pts',(-7.26375799435716,0.74996988957729,4.58495060473737));
#12720=CARTESIAN_POINT('Ctrl Pts',(-7.62294571861381,0.495187693439224,
4.60137479256222));
#12721=CARTESIAN_POINT('Ctrl Pts',(-7.79180148886195,0.0878321179432545,
4.6178157625393));
#12722=CARTESIAN_POINT('Ctrl Pts',(-7.73007153353779,-0.274632525096982,
4.63153055763558));
#12723=CARTESIAN_POINT('Ctrl Pts',(-7.57089063696386,-0.512111859070372,
4.64251171031102));
#12724=CARTESIAN_POINT('Ctrl Pts',(-7.35262771058493,-0.696995379209438,
4.65349879703564));
#12725=CARTESIAN_POINT('Ctrl Pts',(-6.99862347533104,-0.799249420049326,
4.66724321525578));
#12726=CARTESIAN_POINT('Ctrl Pts',(-6.5730502033671,-0.676668689478975,
4.68375532144801));
#12727=CARTESIAN_POINT('Ctrl Pts',(-6.27764603292305,-0.346222659526638,
4.70028617112997));
#12728=CARTESIAN_POINT('Ctrl Pts',(-6.20321862496408,0.0913138303420951,
4.71683637846958));
#12729=CARTESIAN_POINT('Ctrl Pts',(-6.3731989872548,0.501843406155816,4.73340624603523));
#12730=CARTESIAN_POINT('Ctrl Pts',(-6.7359781539714,0.75934304394148,4.74999621871112));
#12731=CARTESIAN_POINT('Ctrl Pts',(-7.18070827957232,0.78438157978822,4.7666066278755));
#12732=CARTESIAN_POINT('Ctrl Pts',(-7.5710873754965,0.568720907705442,4.78323791268823));
#12733=CARTESIAN_POINT('Ctrl Pts',(-7.7871878954453,0.177879522683858,4.79989027648649));
#12734=CARTESIAN_POINT('Ctrl Pts',(-7.76219315364765,-0.268520028593769,
4.81656438241647));
#12735=CARTESIAN_POINT('Ctrl Pts',(-7.50325083995188,-0.633887980333893,
4.83325981631157));
#12736=CARTESIAN_POINT('Ctrl Pts',(-7.08900958601159,-0.805258128798486,
4.84997847660876));
#12737=CARTESIAN_POINT('Ctrl Pts',(-6.64648651499231,-0.730418221478834,
4.86671963489532));
#12738=CARTESIAN_POINT('Ctrl Pts',(-6.31122984273527,-0.430620194746299,
4.88348417172117));
#12739=CARTESIAN_POINT('Ctrl Pts',(-6.22817497301499,-0.14287585295958,
4.89467473489709));
#12740=CARTESIAN_POINT('Ctrl Pts',(-6.22815549748057,0.00192704684477944,
4.9002754633636));
#12741=CARTESIAN_POINT('Ctrl Pts',(-6.18504029502821,0.00193448151638033,
1.00003735833913));
#12742=CARTESIAN_POINT('Ctrl Pts',(-6.18506085287023,0.154785094133507,
1.00594935850175));
#12743=CARTESIAN_POINT('Ctrl Pts',(-6.27276333944073,0.459023202656318,
1.01778085296466));
#12744=CARTESIAN_POINT('Ctrl Pts',(-6.62802047127092,0.776941905279901,
1.03555190416764));
#12745=CARTESIAN_POINT('Ctrl Pts',(-7.09833345900095,0.856671496747452,
1.05334612192011));
#12746=CARTESIAN_POINT('Ctrl Pts',(-7.53984756346967,0.674214010051848,
1.07116357476926));
#12747=CARTESIAN_POINT('Ctrl Pts',(-7.81668484764973,0.283933690087942,
1.08900405680934));
#12748=CARTESIAN_POINT('Ctrl Pts',(-7.84363617288521,-0.194258242749199,
1.10686720694953));
#12749=CARTESIAN_POINT('Ctrl Pts',(-7.6117174721288,-0.614100052993139,
1.12475288155903));
#12750=CARTESIAN_POINT('Ctrl Pts',(-7.19145858739647,-0.846449404226388,
1.14266083536209));
#12751=CARTESIAN_POINT('Ctrl Pts',(-6.71147351063424,-0.819590956705147,
1.16059082409754));
#12752=CARTESIAN_POINT('Ctrl Pts',(-6.31872073476413,-0.541091061200067,
1.17854264946671));
#12753=CARTESIAN_POINT('Ctrl Pts',(-6.16519721681528,-0.170078173925239,
1.19352038967065));
#12754=CARTESIAN_POINT('Ctrl Pts',(-6.1744086284735,0.142017095597367,1.20551337044202));
#12755=CARTESIAN_POINT('Ctrl Pts',(-6.26882012143519,0.439818968973141,
1.21751340794948));
#12756=CARTESIAN_POINT('Ctrl Pts',(-6.53679306581284,0.740104540264321,
1.2325263267041));
#12757=CARTESIAN_POINT('Ctrl Pts',(-7.00162674500001,0.874047532223047,
1.25056268894745));
#12758=CARTESIAN_POINT('Ctrl Pts',(-7.46686569583001,0.740096839109722,
1.26861943195502));
#12759=CARTESIAN_POINT('Ctrl Pts',(-7.78994676609457,0.378704727073858,
1.28669632216987));
#12760=CARTESIAN_POINT('Ctrl Pts',(-7.87129533220736,-0.0996909691720917,
1.30479301011282));
#12761=CARTESIAN_POINT('Ctrl Pts',(-7.68546305982998,-0.548533502869181,
1.32290918478904));
#12762=CARTESIAN_POINT('Ctrl Pts',(-7.2888893757855,-0.830004177694432,
1.34104450291075));
#12763=CARTESIAN_POINT('Ctrl Pts',(-6.80284662879364,-0.857371495441115,
1.35919862600619));
#12764=CARTESIAN_POINT('Ctrl Pts',(-6.37630721910642,-0.62171240423037,
1.37737119834619));
#12765=CARTESIAN_POINT('Ctrl Pts',(-6.14029008944201,-0.194815129798296,
1.39556186131529));
#12766=CARTESIAN_POINT('Ctrl Pts',(-6.1675992442859,0.292692098595048,1.41377024261863));
#12767=CARTESIAN_POINT('Ctrl Pts',(-6.4503620565862,0.691329238623259,1.43199596178485));
#12768=CARTESIAN_POINT('Ctrl Pts',(-6.90229353244458,0.878592492416463,
1.45023864246069));
#12769=CARTESIAN_POINT('Ctrl Pts',(-7.3850203982638,0.796649505790598,1.46849785770109));
#12770=CARTESIAN_POINT('Ctrl Pts',(-7.75048564762091,0.470116177201949,
1.48677326782443));
#12771=CARTESIAN_POINT('Ctrl Pts',(-7.88631090938092,-0.00114003308241335,
1.50506431154639));
#12772=CARTESIAN_POINT('Ctrl Pts',(-7.75049450355181,-0.472989727708301,
1.52337088433291));
#12773=CARTESIAN_POINT('Ctrl Pts',(-7.44516447734219,-0.745614857762243,
1.53863831810871));
#12774=CARTESIAN_POINT('Ctrl Pts',(-7.14185932067798,-0.841789876750141,
1.55086037195908));
#12775=CARTESIAN_POINT('Ctrl Pts',(-6.82363866744145,-0.851230986545527,
1.5630872130319));
#12776=CARTESIAN_POINT('Ctrl Pts',(-6.4617685488527,-0.701448731340242,
1.57769859306773));
#12777=CARTESIAN_POINT('Ctrl Pts',(-6.18876956484561,-0.34076204481659,
1.59470138391594));
#12778=CARTESIAN_POINT('Ctrl Pts',(-6.12396946764894,0.0886308712451369,
1.6110341660673));
#12779=CARTESIAN_POINT('Ctrl Pts',(-6.27258422281589,0.497118933516093,
1.62737718838713));
#12780=CARTESIAN_POINT('Ctrl Pts',(-6.59866814413671,0.784876696180629,
1.64372989468327));
#12781=CARTESIAN_POINT('Ctrl Pts',(-7.02281705661602,0.881754356975332,
1.66009208771515));
#12782=CARTESIAN_POINT('Ctrl Pts',(-7.44212133414031,0.763816074620149,
1.67646326617426));
#12783=CARTESIAN_POINT('Ctrl Pts',(-7.7535740269982,0.459712179182955,1.69284330156785));
#12784=CARTESIAN_POINT('Ctrl Pts',(-7.89729582298658,-0.00309554884323294,
1.71105347450618));
#12785=CARTESIAN_POINT('Ctrl Pts',(-7.74565582599341,-0.527339088652752,
1.73109590677901));
#12786=CARTESIAN_POINT('Ctrl Pts',(-7.26120105934481,-0.875694925054935,
1.75297406892667));
#12787=CARTESIAN_POINT('Ctrl Pts',(-6.71534965504902,-0.852596704401631,
1.77304116487539));
#12788=CARTESIAN_POINT('Ctrl Pts',(-6.32138409450613,-0.56830758518348,
1.79129152330856));
#12789=CARTESIAN_POINT('Ctrl Pts',(-6.13168016009827,-0.174995072057024,
1.80772340676423));
#12790=CARTESIAN_POINT('Ctrl Pts',(-6.15346807946314,0.261805298226859,
1.8241613205225));
#12791=CARTESIAN_POINT('Ctrl Pts',(-6.3814999287675,0.634928357941657,1.84060479295286));
#12792=CARTESIAN_POINT('Ctrl Pts',(-6.76030269950564,0.853656791887009,
1.85705375788615));
#12793=CARTESIAN_POINT('Ctrl Pts',(-7.19789052510478,0.864714230059756,
1.87350701678844));
#12794=CARTESIAN_POINT('Ctrl Pts',(-7.52226056848553,0.698064177431438,
1.88722279945193));
#12795=CARTESIAN_POINT('Ctrl Pts',(-7.71070782550361,0.484061348889512,
1.89819798603134));
#12796=CARTESIAN_POINT('Ctrl Pts',(-7.84108555720893,0.230444159542277,
1.90917447353455));
#12797=CARTESIAN_POINT('Ctrl Pts',(-7.87753262696172,-0.132633185091885,
1.92289532864967));
#12798=CARTESIAN_POINT('Ctrl Pts',(-7.70754420346973,-0.536305861250017,
1.93936662503784));
#12799=CARTESIAN_POINT('Ctrl Pts',(-7.36494164093582,-0.809602048425494,
1.95583772289023));
#12800=CARTESIAN_POINT('Ctrl Pts',(-6.96941379361634,-0.878990673585998,
1.97094063523801));
#12801=CARTESIAN_POINT('Ctrl Pts',(-6.6214605738567,-0.785512528627816,
1.98467314307479));
#12802=CARTESIAN_POINT('Ctrl Pts',(-6.36049958258628,-0.593104694820152,
1.99703284926989));
#12803=CARTESIAN_POINT('Ctrl Pts',(-6.18806293476214,-0.31846173055547,
2.009393865417));
#12804=CARTESIAN_POINT('Ctrl Pts',(-6.12765851408817,0.000201419297515972,
2.02175553044862));
#12805=CARTESIAN_POINT('Ctrl Pts',(-6.18805878567595,0.318766070561102,
2.03411794133265));
#12806=CARTESIAN_POINT('Ctrl Pts',(-6.36052742775184,0.593653877290259,
2.0464809140462));
#12807=CARTESIAN_POINT('Ctrl Pts',(-6.62153479810473,0.785659877107895,
2.05884415784856));
#12808=CARTESIAN_POINT('Ctrl Pts',(-7.03930435057696,0.899103574502222,
2.07532922744145));
#12809=CARTESIAN_POINT('Ctrl Pts',(-7.58335701362722,0.732049936951038,
2.09593354806076));
#12810=CARTESIAN_POINT('Ctrl Pts',(-7.92551787329716,0.139411230229194,
2.1206590672799));
#12811=CARTESIAN_POINT('Ctrl Pts',(-7.77324093952945,-0.526992586217095,
2.14538184010843));
#12812=CARTESIAN_POINT('Ctrl Pts',(-7.2084092233759,-0.912170787733487,
2.17010128170181));
#12813=CARTESIAN_POINT('Ctrl Pts',(-6.53249969066519,-0.810226392153337,
2.19481578239594));
#12814=CARTESIAN_POINT('Ctrl Pts',(-6.1064692514412,-0.275947007217316,
2.21952419869039));
#12815=CARTESIAN_POINT('Ctrl Pts',(-6.15755851138988,0.405302051662446,
2.24422520707067));
#12816=CARTESIAN_POINT('Ctrl Pts',(-6.65820462432343,0.869765062388611,
2.26891757489148));
#12817=CARTESIAN_POINT('Ctrl Pts',(-7.3408453138212,0.869712680842248,2.29360004643675));
#12818=CARTESIAN_POINT('Ctrl Pts',(-7.84099046916954,0.405562883710353,
2.31827138853594));
#12819=CARTESIAN_POINT('Ctrl Pts',(-7.89188859340855,-0.274527300040944,
2.3429303738485));
#12820=CARTESIAN_POINT('Ctrl Pts',(-7.46684950513523,-0.80739148940899,
2.36757578662995));
#12821=CARTESIAN_POINT('Ctrl Pts',(-6.7932369408934,-0.90884115826819,2.39220642377932));
#12822=CARTESIAN_POINT('Ctrl Pts',(-6.23080912069766,-0.525280033465689,
2.41682109261757));
#12823=CARTESIAN_POINT('Ctrl Pts',(-6.07951966246936,0.137978359245954,
2.44141861634764));
#12824=CARTESIAN_POINT('Ctrl Pts',(-6.41950013676486,0.726640754772934,
2.46599782859082));
#12825=CARTESIAN_POINT('Ctrl Pts',(-7.06860259417947,0.926755491531088,
2.49055758358057));
#12826=CARTESIAN_POINT('Ctrl Pts',(-7.68002986417738,0.632179798873464,
2.5150967369546));
#12827=CARTESIAN_POINT('Ctrl Pts',(-7.92764552134961,0.000944522328351112,
2.53961419282274));
#12828=CARTESIAN_POINT('Ctrl Pts',(-7.68005721336133,-0.629669549355358,
2.56410878618908));
#12829=CARTESIAN_POINT('Ctrl Pts',(-7.07019550228192,-0.923123702908933,
2.5885795656002));
#12830=CARTESIAN_POINT('Ctrl Pts',(-6.42429617364977,-0.723912036667828,
2.61302511363373));
#12831=CARTESIAN_POINT('Ctrl Pts',(-6.08649119115101,-0.138517440976113,
2.63744512150446));
#12832=CARTESIAN_POINT('Ctrl Pts',(-6.21223966684041,0.408665861755775,
2.65777140910349));
#12833=CARTESIAN_POINT('Ctrl Pts',(-6.51498330382994,0.709351113648519,
2.674020274529));
#12834=CARTESIAN_POINT('Ctrl Pts',(-6.80735978088213,0.837439867343505,
2.68619945257517));
#12835=CARTESIAN_POINT('Ctrl Pts',(-7.12664566011944,0.849157334778109,
2.6983714927253));
#12836=CARTESIAN_POINT('Ctrl Pts',(-7.42783351180677,0.743878457965117,
2.71053617994053));
#12837=CARTESIAN_POINT('Ctrl Pts',(-7.66951637957178,0.53572864979586,2.72269330897038));
#12838=CARTESIAN_POINT('Ctrl Pts',(-7.81855579145374,0.253955441206058,
2.73484314375331));
#12839=CARTESIAN_POINT('Ctrl Pts',(-7.85400455176983,-0.062539492106813,
2.74698487897661));
#12840=CARTESIAN_POINT('Ctrl Pts',(-7.75818762301745,-0.421432107598265,
2.76114224858493));
#12841=CARTESIAN_POINT('Ctrl Pts',(-7.46987365614386,-0.744902407746362,
2.77730708509788));
#12842=CARTESIAN_POINT('Ctrl Pts',(-7.00137013388183,-0.879557403138088,
2.79547350221892));
#12843=CARTESIAN_POINT('Ctrl Pts',(-6.53382613240907,-0.744802175259395,
2.81362214087364));
#12844=CARTESIAN_POINT('Ctrl Pts',(-6.20983574866432,-0.382182712148995,
2.83175179566087));
#12845=CARTESIAN_POINT('Ctrl Pts',(-6.12857703292412,0.0966500403142058,
2.84986244064629));
#12846=CARTESIAN_POINT('Ctrl Pts',(-6.31430871100684,0.544862222497401,
2.86795349734992));
#12847=CARTESIAN_POINT('Ctrl Pts',(-6.70959717985322,0.825242975432329,
2.88602481111419));
#12848=CARTESIAN_POINT('Ctrl Pts',(-7.19296888464305,0.852302747612439,
2.90407573088816));
#12849=CARTESIAN_POINT('Ctrl Pts',(-7.6160819344623,0.618348268313813,2.92210658574007));
#12850=CARTESIAN_POINT('Ctrl Pts',(-7.84982079765454,0.195559912762412,
2.94011563526226));
#12851=CARTESIAN_POINT('Ctrl Pts',(-7.82237000115257,-0.286026340065306,
2.95810576365756));
#12852=CARTESIAN_POINT('Ctrl Pts',(-7.54353880028185,-0.678962954634159,
2.97607295385774));
#12853=CARTESIAN_POINT('Ctrl Pts',(-7.09889613896107,-0.863059411748946,
2.99401870845086));
#12854=CARTESIAN_POINT('Ctrl Pts',(-6.62504791383588,-0.782464854277864,
3.01194258453785));
#12855=CARTESIAN_POINT('Ctrl Pts',(-6.26714694908666,-0.462504395091709,
3.02984438133514));
#12856=CARTESIAN_POINT('Ctrl Pts',(-6.13450086477898,-0.0017428437012401,
3.04772383986694));
#12857=CARTESIAN_POINT('Ctrl Pts',(-6.26715807301811,0.458389157575083,
3.06558074068058));
#12858=CARTESIAN_POINT('Ctrl Pts',(-6.62383159683867,0.777010504229039,
3.08341486755061));
#12859=CARTESIAN_POINT('Ctrl Pts',(-7.09474387207995,0.856931067075294,
3.10122601821375));
#12860=CARTESIAN_POINT('Ctrl Pts',(-7.53542180806767,0.674300001519429,
3.11901400258171));
#12861=CARTESIAN_POINT('Ctrl Pts',(-7.81102536987665,0.285718970191242,
3.1367786406439));
#12862=CARTESIAN_POINT('Ctrl Pts',(-7.83761192611158,-0.189300816311006,
3.15451976374402));
#12863=CARTESIAN_POINT('Ctrl Pts',(-7.60770460153743,-0.605099341888002,
3.1722372169101));
#12864=CARTESIAN_POINT('Ctrl Pts',(-7.192377909984,-0.834537764149841,3.18993085280259));
#12865=CARTESIAN_POINT('Ctrl Pts',(-6.71928442386195,-0.807877081114413,
3.20760053887308));
#12866=CARTESIAN_POINT('Ctrl Pts',(-6.33341662752147,-0.533975589038894,
3.22524615138231));
#12867=CARTESIAN_POINT('Ctrl Pts',(-6.1526663682926,-0.0973624004398561,
3.24286758015074));
#12868=CARTESIAN_POINT('Ctrl Pts',(-6.23180408134589,0.367850412115243,
3.26046472470488));
#12869=CARTESIAN_POINT('Ctrl Pts',(-6.5458840541067,0.7191652253215,3.27803749683208));
#12870=CARTESIAN_POINT('Ctrl Pts',(-6.99810294271046,0.849349265206921,
3.29558582036997));
#12871=CARTESIAN_POINT('Ctrl Pts',(-7.44963689661624,0.719166284808225,
3.31310962945538));
#12872=CARTESIAN_POINT('Ctrl Pts',(-7.76226017562776,0.369198513354485,
3.33060887092856));
#12873=CARTESIAN_POINT('Ctrl Pts',(-7.84066094364821,-0.0928017396707875,
3.34808350242358));
#12874=CARTESIAN_POINT('Ctrl Pts',(-7.66149885418233,-0.525088884595006,
3.3655334936625));
#12875=CARTESIAN_POINT('Ctrl Pts',(-7.28034773305643,-0.79541391783641,
3.38295882562499));
#12876=CARTESIAN_POINT('Ctrl Pts',(-6.81445718631064,-0.821483139569074,
3.40035949040031));
#12877=CARTESIAN_POINT('Ctrl Pts',(-6.40668765829451,-0.59600943840361,
3.41773549312221));
#12878=CARTESIAN_POINT('Ctrl Pts',(-6.18169584214414,-0.188728419605418,
3.43508684584969));
#12879=CARTESIAN_POINT('Ctrl Pts',(-6.20784514290506,0.275165281873529,
3.45241358192968));
#12880=CARTESIAN_POINT('Ctrl Pts',(-6.47639639507144,0.653507341417247,
3.46971572219518));
#12881=CARTESIAN_POINT('Ctrl Pts',(-6.90449682661278,0.830715021230648,
3.48699334992386));
#12882=CARTESIAN_POINT('Ctrl Pts',(-7.36054265068983,0.75312759896658,3.50424644156099));
#12883=CARTESIAN_POINT('Ctrl Pts',(-7.70507323679672,0.445177926714059,
3.52147524374292));
#12884=CARTESIAN_POINT('Ctrl Pts',(-7.81119433678745,0.075752404018898,
3.53581204983664));
#12885=CARTESIAN_POINT('Ctrl Pts',(-7.76904314299935,-0.219543515671938,
3.54726986688073));
#12886=CARTESIAN_POINT('Ctrl Pts',(-7.64765861917188,-0.491844914406571,
3.55871960593793));
#12887=CARTESIAN_POINT('Ctrl Pts',(-7.36203942815138,-0.747244560961086,
3.57301619085879));
#12888=CARTESIAN_POINT('Ctrl Pts',(-6.90878559141423,-0.824346342944035,
3.59014821043938));
#12889=CARTESIAN_POINT('Ctrl Pts',(-6.5325070262611,-0.667772572877197,
3.60535557378859));
#12890=CARTESIAN_POINT('Ctrl Pts',(-6.30530616111317,-0.403207986958227,
3.61864694286058));
#12891=CARTESIAN_POINT('Ctrl Pts',(-6.20656869022908,-0.121503914492411,
3.63002891106073));
#12892=CARTESIAN_POINT('Ctrl Pts',(-6.21786904271036,0.17661120472348,3.64140045843225));
#12893=CARTESIAN_POINT('Ctrl Pts',(-6.33697049241504,0.449785070539879,
3.65276160378139));
#12894=CARTESIAN_POINT('Ctrl Pts',(-6.54761646387189,0.660239824218537,
3.66411237271902));
#12895=CARTESIAN_POINT('Ctrl Pts',(-6.82024360477912,0.779264913606105,
3.67545286820712));
#12896=CARTESIAN_POINT('Ctrl Pts',(-7.11728136597602,0.790317129746521,
3.68678318085792));
#12897=CARTESIAN_POINT('Ctrl Pts',(-7.33526250184263,0.714001102786347,
3.69558769336262));
#12898=CARTESIAN_POINT('Ctrl Pts',(-7.52460478021158,0.588335445521869,
3.7043869786929));
#12899=CARTESIAN_POINT('Ctrl Pts',(-7.70168747930115,0.392944569857713,
3.71443734764326));
#12900=CARTESIAN_POINT('Ctrl Pts',(-7.80988273301986,0.0422429930341788,
3.72824225157302));
#12901=CARTESIAN_POINT('Ctrl Pts',(-7.72727513305559,-0.366328708453495,
3.74391125197574));
#12902=CARTESIAN_POINT('Ctrl Pts',(-7.43666554118108,-0.691696849479157,
3.76018685693119));
#12903=CARTESIAN_POINT('Ctrl Pts',(-7.00161691448238,-0.816915579528899,
3.77706653049292));
#12904=CARTESIAN_POINT('Ctrl Pts',(-6.56733396055601,-0.691682810651421,
3.79392454460657));
#12905=CARTESIAN_POINT('Ctrl Pts',(-6.26654562765578,-0.3550205123833,3.81076115841936));
#12906=CARTESIAN_POINT('Ctrl Pts',(-6.1911325553665,0.0895827193733467,
3.82757667281065));
#12907=CARTESIAN_POINT('Ctrl Pts',(-6.36350946096962,0.50548282085585,3.84437132520021));
#12908=CARTESIAN_POINT('Ctrl Pts',(-6.73047124123842,0.766010242524385,
3.86114554454008));
#12909=CARTESIAN_POINT('Ctrl Pts',(-7.12901368034643,0.787746171743655,
3.87603784194693));
#12910=CARTESIAN_POINT('Ctrl Pts',(-7.44190892966169,0.650845344649784,
3.88905532446545));
#12911=CARTESIAN_POINT('Ctrl Pts',(-7.64878134275722,0.444189022830509,
3.90020462760315));
#12912=CARTESIAN_POINT('Ctrl Pts',(-7.76553306778079,0.176269133820623,
3.91134511925484));
#12913=CARTESIAN_POINT('Ctrl Pts',(-7.77653094523285,-0.115552363536951,
3.92247714568019));
#12914=CARTESIAN_POINT('Ctrl Pts',(-7.68006611264172,-0.390854840429437,
3.9336006136539));
#12915=CARTESIAN_POINT('Ctrl Pts',(-7.48992306377386,-0.612073383815134,
3.94471576165104));
#12916=CARTESIAN_POINT('Ctrl Pts',(-7.23237165848447,-0.747663663403516,
3.95582259199976));
#12917=CARTESIAN_POINT('Ctrl Pts',(-6.84646473121294,-0.792403433674334,
3.97062077929395));
#12918=CARTESIAN_POINT('Ctrl Pts',(-6.3864410792178,-0.571475980182002,
3.98909889576364));
#12919=CARTESIAN_POINT('Ctrl Pts',(-6.16238496201624,-0.00115785824039473,
4.01124054191812));
#12920=CARTESIAN_POINT('Ctrl Pts',(-6.3862304211917,0.567803406777749,4.03335240929006));
#12921=CARTESIAN_POINT('Ctrl Pts',(-6.93635510725266,0.832684234789182,
4.05543432814072));
#12922=CARTESIAN_POINT('Ctrl Pts',(-7.51909126085599,0.652689650771393,
4.07748779641409));
#12923=CARTESIAN_POINT('Ctrl Pts',(-7.82352412968288,0.125343566686662,
4.09951350361257));
#12924=CARTESIAN_POINT('Ctrl Pts',(-7.68796000136869,-0.468110630686831,
4.12151270501089));
#12925=CARTESIAN_POINT('Ctrl Pts',(-7.2418525938744,-0.771426362219948,
4.14104449245175));
#12926=CARTESIAN_POINT('Ctrl Pts',(-6.7873808143172,-0.758570879140142,
4.15811957803281));
#12927=CARTESIAN_POINT('Ctrl Pts',(-6.45084731947709,-0.564693301253677,
4.1727448719699));
#12928=CARTESIAN_POINT('Ctrl Pts',(-6.24818669107861,-0.232820084937952,
4.18735958652774));
#12929=CARTESIAN_POINT('Ctrl Pts',(-6.22869241803636,0.154912462764796,
4.20196415138622));
#12930=CARTESIAN_POINT('Ctrl Pts',(-6.39729009617743,0.504573285610341,
4.21655860239769));
#12931=CARTESIAN_POINT('Ctrl Pts',(-6.68600830745319,0.7119144340067,4.22993002217742));
#12932=CARTESIAN_POINT('Ctrl Pts',(-6.99915603726572,0.770953989010427,
4.24207743095502));
#12933=CARTESIAN_POINT('Ctrl Pts',(-7.28083374176742,0.717756806009324,
4.25300578778819));
#12934=CARTESIAN_POINT('Ctrl Pts',(-7.52332570145096,0.565265639900522,
4.26392915087842));
#12935=CARTESIAN_POINT('Ctrl Pts',(-7.69361125094384,0.334758364883805,
4.27484799782803));
#12936=CARTESIAN_POINT('Ctrl Pts',(-7.76721204522818,0.0585123291627315,
4.28576249660097));
#12937=CARTESIAN_POINT('Ctrl Pts',(-7.72563755456501,-0.321492167904461,
4.30030880645676));
#12938=CARTESIAN_POINT('Ctrl Pts',(-7.47577070976408,-0.634729906167413,
4.31484910788061));
#12939=CARTESIAN_POINT('Ctrl Pts',(-7.11494082441407,-0.75964778831911,
4.32937923018361));
#12940=CARTESIAN_POINT('Ctrl Pts',(-6.82977343242683,-0.749363011330386,
4.3402736097982));
#12941=CARTESIAN_POINT('Ctrl Pts',(-6.5678367429364,-0.63491734918943,4.35116416567639));
#12942=CARTESIAN_POINT('Ctrl Pts',(-6.36591104875818,-0.433096850888867,
4.36205133937433));
#12943=CARTESIAN_POINT('Ctrl Pts',(-6.25181603734438,-0.171382362262575,
4.37293523607869));
#12944=CARTESIAN_POINT('Ctrl Pts',(-6.24105003663889,0.113834567019171,
4.38381579035452));
#12945=CARTESIAN_POINT('Ctrl Pts',(-6.33542564510066,0.383034418620386,
4.39469364740737));
#12946=CARTESIAN_POINT('Ctrl Pts',(-6.55230017515376,0.63552240326747,4.40738028050328));
#12947=CARTESIAN_POINT('Ctrl Pts',(-6.91099640381501,0.784687258636925,
4.4218763046563));
#12948=CARTESIAN_POINT('Ctrl Pts',(-7.34212240019886,0.711207343436876,
4.43817956917959));
#12949=CARTESIAN_POINT('Ctrl Pts',(-7.66784503795017,0.420122820836888,
4.45447719499099));
#12950=CARTESIAN_POINT('Ctrl Pts',(-7.78880772644369,0.000301349021138111,
4.4707704498999));
#12951=CARTESIAN_POINT('Ctrl Pts',(-7.667877587161,-0.419341085827839,4.48705960232271));
#12952=CARTESIAN_POINT('Ctrl Pts',(-7.34230267069937,-0.710297515575184,
4.50334535553822));
#12953=CARTESIAN_POINT('Ctrl Pts',(-6.91190437925101,-0.783412060401462,
4.51962819595119));
#12954=CARTESIAN_POINT('Ctrl Pts',(-6.50863628128277,-0.616365790333621,
4.53590870397414));
#12955=CARTESIAN_POINT('Ctrl Pts',(-6.25607982849799,-0.260409693527577,
4.5521874093325));
#12956=CARTESIAN_POINT('Ctrl Pts',(-6.23161283377708,0.175321606389228,
4.56846487082594));
#12957=CARTESIAN_POINT('Ctrl Pts',(-6.44271176828563,0.557262980844724,
4.58474160682034));
#12958=CARTESIAN_POINT('Ctrl Pts',(-6.82464434492978,0.768358222162331,
4.60101821545767));
#12959=CARTESIAN_POINT('Ctrl Pts',(-7.26037536186215,0.743876395320755,
4.61729512256828));
#12960=CARTESIAN_POINT('Ctrl Pts',(-7.61626704964913,0.491357056997004,
4.63357315010908));
#12961=CARTESIAN_POINT('Ctrl Pts',(-7.78338185515668,0.0880536646158774,
4.64985222966985));
#12962=CARTESIAN_POINT('Ctrl Pts',(-7.72227904989592,-0.270456594079558,
4.66342067449138));
#12963=CARTESIAN_POINT('Ctrl Pts',(-7.56494361675605,-0.505166038725783,
4.67427498609028));
#12964=CARTESIAN_POINT('Ctrl Pts',(-7.34931051926875,-0.687808815183051,
4.68513021846502));
#12965=CARTESIAN_POINT('Ctrl Pts',(-6.99978283745156,-0.788718364067694,
4.69870330867372));
#12966=CARTESIAN_POINT('Ctrl Pts',(-6.58001528872106,-0.667748618933984,
4.71499348628701));
#12967=CARTESIAN_POINT('Ctrl Pts',(-6.28892712013077,-0.342052929566312,
4.7312881611743));
#12968=CARTESIAN_POINT('Ctrl Pts',(-6.21569469059752,0.0887734809755611,
4.74758724186428));
#12969=CARTESIAN_POINT('Ctrl Pts',(-6.38296454904747,0.492623142936048,
4.76389156558651));
#12970=CARTESIAN_POINT('Ctrl Pts',(-6.739578169164,0.745682782278417,4.78020152499504));
#12971=CARTESIAN_POINT('Ctrl Pts',(-7.17633951141972,0.770218713454861,
4.79651776702086));
#12972=CARTESIAN_POINT('Ctrl Pts',(-7.55937071328772,0.558553081416467,
4.81284069537888));
#12973=CARTESIAN_POINT('Ctrl Pts',(-7.77118600830977,0.175328612777807,
4.8291711200582));
#12974=CARTESIAN_POINT('Ctrl Pts',(-7.74663968736165,-0.261977048857528,
4.84550903765717));
#12975=CARTESIAN_POINT('Ctrl Pts',(-7.49310132503884,-0.61959334356644,
4.86185626860575));
#12976=CARTESIAN_POINT('Ctrl Pts',(-7.08792565192062,-0.787152269199519,
4.87821065600015));
#12977=CARTESIAN_POINT('Ctrl Pts',(-6.65545106666535,-0.713968083417749,
4.89457308734717));
#12978=CARTESIAN_POINT('Ctrl Pts',(-6.32807722541735,-0.421152088596462,
4.910946967621));
#12979=CARTESIAN_POINT('Ctrl Pts',(-6.24702100712985,-0.140397334609587,
4.92186764777286));
#12980=CARTESIAN_POINT('Ctrl Pts',(-6.24700200535915,0.000883075965957197,
4.92733213238152));
#12981=CARTESIAN_POINT('Ctrl Pts',(-6.20000025990999,0.00193246945643844,
1.00003735833913));
#12982=CARTESIAN_POINT('Ctrl Pts',(-6.20002044487095,0.15201065585541,1.00584212579936));
#12983=CARTESIAN_POINT('Ctrl Pts',(-6.28611355781982,0.450654413607575,
1.01745595262984));
#12984=CARTESIAN_POINT('Ctrl Pts',(-6.63487773043299,0.762776896374944,
1.0349026678303));
#12985=CARTESIAN_POINT('Ctrl Pts',(-7.09661480461016,0.841046944166038,
1.05237210147879));
#12986=CARTESIAN_POINT('Ctrl Pts',(-7.5301000809641,0.66191148032223,1.06986555847399));
#12987=CARTESIAN_POINT('Ctrl Pts',(-7.8019176387512,0.278705057923738,1.08738232429735));
#12988=CARTESIAN_POINT('Ctrl Pts',(-7.82838413701279,-0.19084760704926,
1.10492270302733));
#12989=CARTESIAN_POINT('Ctrl Pts',(-7.60064075566285,-0.603137091155931,
1.12248646715818));
#12990=CARTESIAN_POINT('Ctrl Pts',(-7.1879122444388,-0.831327694844811,
1.1400736154085));
#12991=CARTESIAN_POINT('Ctrl Pts',(-6.71648331627183,-0.804952825733149,
1.15768402928987));
#12992=CARTESIAN_POINT('Ctrl Pts',(-6.33069129380762,-0.53139586788873,
1.17531762920689));
#12993=CARTESIAN_POINT('Ctrl Pts',(-6.17986938434826,-0.166924530929506,
1.19003152205635));
#12994=CARTESIAN_POINT('Ctrl Pts',(-6.18891827393114,0.139694417819641,
1.20181411747366));
#12995=CARTESIAN_POINT('Ctrl Pts',(-6.28167759636603,0.432287479563812,
1.21360434390419));
#12996=CARTESIAN_POINT('Ctrl Pts',(-6.54498491257115,0.727352514001043,
1.22835639528026));
#12997=CARTESIAN_POINT('Ctrl Pts',(-7.00178799837524,0.858989074734809,
1.2460815491715));
#12998=CARTESIAN_POINT('Ctrl Pts',(-7.45905640505002,0.727341633611197,
1.2638292469814));
#12999=CARTESIAN_POINT('Ctrl Pts',(-7.77665281049733,0.372097321399229,
1.28159932797245));
#13000=CARTESIAN_POINT('Ctrl Pts',(-7.85663990835041,-0.0982374580424732,
1.29939162334549));
#13001=CARTESIAN_POINT('Ctrl Pts',(-7.67391806687674,-0.539592338752092,
1.31720595246947));
#13002=CARTESIAN_POINT('Ctrl Pts',(-7.28390423314539,-0.816419475206943,
1.33504212338853));
#13003=CARTESIAN_POINT('Ctrl Pts',(-6.80581165670056,-0.843349744908527,
1.35289993632842));
#13004=CARTESIAN_POINT('Ctrl Pts',(-6.38616737126169,-0.61151281975725,
1.37077917836497));
#13005=CARTESIAN_POINT('Ctrl Pts',(-6.15391471330266,-0.191448545046746,
1.38867962991899));
#13006=CARTESIAN_POINT('Ctrl Pts',(-6.18078031189829,0.288356063072798,
1.40660105660474));
#13007=CARTESIAN_POINT('Ctrl Pts',(-6.45912099114284,0.680780452257456,
1.42454321935777));
#13008=CARTESIAN_POINT('Ctrl Pts',(-6.90408886634936,0.865172061566579,
1.44250586618275));
#13009=CARTESIAN_POINT('Ctrl Pts',(-7.37948719351768,0.784486199243698,
1.46048873474343));
#13010=CARTESIAN_POINT('Ctrl Pts',(-7.73949168252554,0.462850086060547,
1.47849155669373));
#13011=CARTESIAN_POINT('Ctrl Pts',(-7.87332738631526,-0.0014557841833066,
1.49651404939771));
#13012=CARTESIAN_POINT('Ctrl Pts',(-7.73949699110486,-0.466462821459191,
1.51455592727214));
#13013=CARTESIAN_POINT('Ctrl Pts',(-7.43853082628792,-0.735208997602771,
1.52960672657187));
#13014=CARTESIAN_POINT('Ctrl Pts',(-7.13950426621928,-0.830029799823059,
1.5416567556677));
#13015=CARTESIAN_POINT('Ctrl Pts',(-6.82573429908325,-0.839341203501555,
1.55371299076107));
#13016=CARTESIAN_POINT('Ctrl Pts',(-6.46884268588545,-0.691631510671627,
1.56812451918729));
#13017=CARTESIAN_POINT('Ctrl Pts',(-6.19953260950331,-0.335836989319061,
1.58489796930832));
#13018=CARTESIAN_POINT('Ctrl Pts',(-6.13558329245919,0.087838843174565,
1.60101457637617));
#13019=CARTESIAN_POINT('Ctrl Pts',(-6.28224419701691,0.490989051876738,
1.61714503893002));
#13020=CARTESIAN_POINT('Ctrl Pts',(-6.60413478737033,0.775061465279082,
1.63328911262099));
#13021=CARTESIAN_POINT('Ctrl Pts',(-7.02294084448011,0.870730250827747,
1.64944654818199));
#13022=CARTESIAN_POINT('Ctrl Pts',(-7.43707348216018,0.754258049077075,
1.66561709103637));
#13023=CARTESIAN_POINT('Ctrl Pts',(-7.74477169774561,0.453838654047166,
1.68180048156974));
#13024=CARTESIAN_POINT('Ctrl Pts',(-7.88680288613318,-0.003482702933719,
1.69979600813884));
#13025=CARTESIAN_POINT('Ctrl Pts',(-7.73694295256561,-0.521688074393446,
1.71960864643413));
#13026=CARTESIAN_POINT('Ctrl Pts',(-7.2579246797109,-0.866176668338957,
1.74124367709995));
#13027=CARTESIAN_POINT('Ctrl Pts',(-6.71798257071652,-0.843361624137061,
1.76109465157299));
#13028=CARTESIAN_POINT('Ctrl Pts',(-6.32813840204838,-0.562067108424238,
1.779155502939));
#13029=CARTESIAN_POINT('Ctrl Pts',(-6.1403602470473,-0.172779460138823,
1.79542117132473));
#13030=CARTESIAN_POINT('Ctrl Pts',(-6.16191594592092,0.259681676239064,
1.81169744765855));
#13031=CARTESIAN_POINT('Ctrl Pts',(-6.38773509477738,0.629211178523826,
1.82798403284572));
#13032=CARTESIAN_POINT('Ctrl Pts',(-6.76298297690006,0.845905336791279,
1.84428062449289));
#13033=CARTESIAN_POINT('Ctrl Pts',(-7.1966047520639,0.856877177797125,1.86058691436274));
#13034=CARTESIAN_POINT('Ctrl Pts',(-7.51813159987616,0.691704323104765,
1.87418331464002));
#13035=CARTESIAN_POINT('Ctrl Pts',(-7.70496340534196,0.479537214773933,
1.88506497141452));
#13036=CARTESIAN_POINT('Ctrl Pts',(-7.834243376472,0.228058843588403,1.89594960161061));
#13037=CARTESIAN_POINT('Ctrl Pts',(-7.87040214071621,-0.132058080538115,
1.90956086256863));
#13038=CARTESIAN_POINT('Ctrl Pts',(-7.70176729712619,-0.532544739489079,
1.92590281458038));
#13039=CARTESIAN_POINT('Ctrl Pts',(-7.3617541753632,-0.803795766305812,
1.94225288140178));
#13040=CARTESIAN_POINT('Ctrl Pts',(-6.96910081682361,-0.872691342258758,
1.95724758038991));
#13041=CARTESIAN_POINT('Ctrl Pts',(-6.62358365553027,-0.779878922686934,
1.97088456464667));
#13042=CARTESIAN_POINT('Ctrl Pts',(-6.36438571820951,-0.588772954661729,
1.98316190508021));
#13043=CARTESIAN_POINT('Ctrl Pts',(-6.19306544459119,-0.315928048614165,
1.99544316011942));
#13044=CARTESIAN_POINT('Ctrl Pts',(-6.13303928680132,0.000731296674565001,
2.00772818860116));
#13045=CARTESIAN_POINT('Ctrl Pts',(-6.19306246181983,0.31737131710264,2.02001684693935));
#13046=CARTESIAN_POINT('Ctrl Pts',(-6.36452596264878,0.590662777058206,
2.03230899246722));
#13047=CARTESIAN_POINT('Ctrl Pts',(-6.62407285476001,0.781608449704824,
2.04460448181281));
#13048=CARTESIAN_POINT('Ctrl Pts',(-7.03960726862712,0.894452101215339,
2.06100273047082));
#13049=CARTESIAN_POINT('Ctrl Pts',(-7.58098213708746,0.728278840923384,
2.08150817561209));
#13050=CARTESIAN_POINT('Ctrl Pts',(-7.9216670182819,0.138324035331395,2.10612575173056));
#13051=CARTESIAN_POINT('Ctrl Pts',(-7.77006105183817,-0.525438678362505,
2.13075319116009));
#13052=CARTESIAN_POINT('Ctrl Pts',(-7.20723620509449,-0.909325593088126,
2.15538930422495));
#13053=CARTESIAN_POINT('Ctrl Pts',(-6.53333888373858,-0.807749099412924,
2.18003289797092));
#13054=CARTESIAN_POINT('Ctrl Pts',(-6.1083188432114,-0.274839326778277,
2.204682767912));
#13055=CARTESIAN_POINT('Ctrl Pts',(-6.15924265883207,0.405062095085805,
2.22933770998693));
#13056=CARTESIAN_POINT('Ctrl Pts',(-6.65910391363797,0.868885188693027,
2.25399651054932));
#13057=CARTESIAN_POINT('Ctrl Pts',(-7.34108037988483,0.868897827671466,
2.2786579570982));
#13058=CARTESIAN_POINT('Ctrl Pts',(-7.84103724749041,0.405011680967366,
2.30332083156262));
#13059=CARTESIAN_POINT('Ctrl Pts',(-7.89200269882987,-0.275103355231245,
2.32798391722886));
#13060=CARTESIAN_POINT('Ctrl Pts',(-7.46677961363602,-0.808302976870588,
2.35264599503351));
#13061=CARTESIAN_POINT('Ctrl Pts',(-6.79246102077101,-0.909925026569516,
2.37730584883283));
#13062=CARTESIAN_POINT('Ctrl Pts',(-6.22911235514946,-0.525814889228737,
2.40196226239673));
#13063=CARTESIAN_POINT('Ctrl Pts',(-6.07744456821118,0.138809074175696,
2.42661402385257));
#13064=CARTESIAN_POINT('Ctrl Pts',(-6.41824880300263,0.729027866722014,
2.45125992491537));
#13065=CARTESIAN_POINT('Ctrl Pts',(-7.06934122876124,0.929824149026898,
2.47589876067858));
#13066=CARTESIAN_POINT('Ctrl Pts',(-7.68299796183915,0.634246527935802,
2.50052933613646));
#13067=CARTESIAN_POINT('Ctrl Pts',(-7.93168967879738,0.000445263131447748,
2.52515045678013));
#13068=CARTESIAN_POINT('Ctrl Pts',(-7.68302213647328,-0.633094458923734,
2.54976094441856));
#13069=CARTESIAN_POINT('Ctrl Pts',(-7.07007700890629,-0.928102101680422,
2.57435962067245));
#13070=CARTESIAN_POINT('Ctrl Pts',(-6.42054771123064,-0.727833461900544,
2.59894532553828));
#13071=CARTESIAN_POINT('Ctrl Pts',(-6.08063030273252,-0.138905152375385,
2.62351690334527));
#13072=CARTESIAN_POINT('Ctrl Pts',(-6.20716604633801,0.411896009844242,
2.64398049630671));
#13073=CARTESIAN_POINT('Ctrl Pts',(-6.51199774209192,0.714676452673333,
2.66034317170459));
#13074=CARTESIAN_POINT('Ctrl Pts',(-6.80647130896726,0.843685013671235,
2.67261094147259));
#13075=CARTESIAN_POINT('Ctrl Pts',(-7.12812476587158,0.855502087711664,
2.68487433317324));
#13076=CARTESIAN_POINT('Ctrl Pts',(-7.43161948042588,0.749419002627999,
2.69713320958533));
#13077=CARTESIAN_POINT('Ctrl Pts',(-7.67521904640705,0.539636596661724,
2.7093874343511));
#13078=CARTESIAN_POINT('Ctrl Pts',(-7.82547325176268,0.255576344693996,
2.72163687040038));
#13079=CARTESIAN_POINT('Ctrl Pts',(-7.86123160253771,-0.0635635909156293,
2.73388138286896));
#13080=CARTESIAN_POINT('Ctrl Pts',(-7.76460027897753,-0.425533717492343,
2.74816074914963));
#13081=CARTESIAN_POINT('Ctrl Pts',(-7.47374360660769,-0.751894656156828,
2.76447137187111));
#13082=CARTESIAN_POINT('Ctrl Pts',(-7.00091436223893,-0.88782428734477,
2.78280870439184));
#13083=CARTESIAN_POINT('Ctrl Pts',(-6.52888862282209,-0.751805319722163,
2.80113347394993));
#13084=CARTESIAN_POINT('Ctrl Pts',(-6.2016684053735,-0.385612928895403,
2.81944525307317));
#13085=CARTESIAN_POINT('Ctrl Pts',(-6.11955382035284,0.0981170754742554,
2.83774361225262));
#13086=CARTESIAN_POINT('Ctrl Pts',(-6.30722625617569,0.551073055321834,
2.85602813457377));
#13087=CARTESIAN_POINT('Ctrl Pts',(-6.70680747045044,0.834525970819447,
2.87429840546262));
#13088=CARTESIAN_POINT('Ctrl Pts',(-7.19559869716282,0.861909407171868,
2.8925540164347));
#13089=CARTESIAN_POINT('Ctrl Pts',(-7.62360216624703,0.625277985438662,
2.91079457296321));
#13090=CARTESIAN_POINT('Ctrl Pts',(-7.86012925287909,0.197486531354187,
2.92901967711976));
#13091=CARTESIAN_POINT('Ctrl Pts',(-7.83237012712838,-0.289941720567784,
2.94722894753945));
#13092=CARTESIAN_POINT('Ctrl Pts',(-7.55008001741224,-0.687784692046307,
2.96542200407487));
#13093=CARTESIAN_POINT('Ctrl Pts',(-7.09977586824996,-0.874247976731781,
2.98359847915852));
#13094=CARTESIAN_POINT('Ctrl Pts',(-6.61974323779859,-0.792623075615972,
3.00175800933));
#13095=CARTESIAN_POINT('Ctrl Pts',(-6.257058130519,-0.468413543112272,3.0199002388146));
#13096=CARTESIAN_POINT('Ctrl Pts',(-6.12258713457564,-0.00138700255432796,
3.03802482606703));
#13097=CARTESIAN_POINT('Ctrl Pts',(-6.25706727378645,0.465139317147603,
3.05613142853581));
#13098=CARTESIAN_POINT('Ctrl Pts',(-6.61877666867083,0.788285032559405,
3.07421972093098));
#13099=CARTESIAN_POINT('Ctrl Pts',(-7.09647607914372,0.869376408975484,
3.09228937996591));
#13100=CARTESIAN_POINT('Ctrl Pts',(-7.54362920385282,0.68408153123717,3.11034009649877));
#13101=CARTESIAN_POINT('Ctrl Pts',(-7.82336210739947,0.28970919078182,3.12837156650594));
#13102=CARTESIAN_POINT('Ctrl Pts',(-7.85036951729978,-0.192518648808231,
3.1463834953635));
#13103=CARTESIAN_POINT('Ctrl Pts',(-7.61693284376151,-0.614735291409423,
3.16437560200786));
#13104=CARTESIAN_POINT('Ctrl Pts',(-7.19511476226595,-0.847778676228102,
3.18234760781168));
#13105=CARTESIAN_POINT('Ctrl Pts',(-6.7145098999882,-0.820710857786535,
3.20029925009486));
#13106=CARTESIAN_POINT('Ctrl Pts',(-6.32242256217712,-0.542413764760527,
3.21823027098919));
#13107=CARTESIAN_POINT('Ctrl Pts',(-6.13871066850024,-0.098686345015634,
3.23614042632575));
#13108=CARTESIAN_POINT('Ctrl Pts',(-6.21914065946509,0.374211025419683,
3.25402947870679));
#13109=CARTESIAN_POINT('Ctrl Pts',(-6.53845875539302,0.731406338297415,
3.27189720144838));
#13110=CARTESIAN_POINT('Ctrl Pts',(-6.99831755296742,0.863804065639348,
3.2897433804432));
#13111=CARTESIAN_POINT('Ctrl Pts',(-7.45757029965599,0.731409466469204,
3.30756780748229));
#13112=CARTESIAN_POINT('Ctrl Pts',(-7.77559982146972,0.37540881511312,3.32537028850097));
#13113=CARTESIAN_POINT('Ctrl Pts',(-7.85537931424834,-0.094642652826617,
3.34315063708933));
#13114=CARTESIAN_POINT('Ctrl Pts',(-7.67307624395954,-0.534539169893111,
3.36090867961867));
#13115=CARTESIAN_POINT('Ctrl Pts',(-7.28516805861167,-0.809670332991083,
3.37864425091963));
#13116=CARTESIAN_POINT('Ctrl Pts',(-6.81094328129299,-0.836216654728318,
3.39635719733567));
#13117=CARTESIAN_POINT('Ctrl Pts',(-6.39581795219668,-0.606687244699812,
3.41404737686194));
#13118=CARTESIAN_POINT('Ctrl Pts',(-6.16673282986248,-0.192016386472062,
3.43171465630725));
#13119=CARTESIAN_POINT('Ctrl Pts',(-6.19335105955753,0.280356102113162,
3.44935891493111));
#13120=CARTESIAN_POINT('Ctrl Pts',(-6.46683379484748,0.665660108445628,
3.46698004190314));
#13121=CARTESIAN_POINT('Ctrl Pts',(-6.90284795213186,0.846152102600437,
3.48457793824716));
#13122=CARTESIAN_POINT('Ctrl Pts',(-7.36737219772646,0.767129205800447,
3.50215251490095));
#13123=CARTESIAN_POINT('Ctrl Pts',(-7.71834143496065,0.453434200086869,
3.51970369457236));
#13124=CARTESIAN_POINT('Ctrl Pts',(-7.82645846631761,0.077080609195679,
3.53431012488451));
#13125=CARTESIAN_POINT('Ctrl Pts',(-7.78351602643939,-0.223766099777631,
3.54598350983127));
#13126=CARTESIAN_POINT('Ctrl Pts',(-7.65984666406284,-0.501195016191524,
3.55764904771478));
#13127=CARTESIAN_POINT('Ctrl Pts',(-7.36883520137935,-0.761421141511966,
3.57221624328425));
#13128=CARTESIAN_POINT('Ctrl Pts',(-6.90699782821215,-0.839986918687281,
3.58967328199228));
#13129=CARTESIAN_POINT('Ctrl Pts',(-6.5235772119384,-0.680444831465126,
3.60516965595896));
#13130=CARTESIAN_POINT('Ctrl Pts',(-6.29205860881578,-0.410854643842501,
3.6187136684483));
#13131=CARTESIAN_POINT('Ctrl Pts',(-6.19144251696091,-0.123792268925567,
3.63031232027941));
#13132=CARTESIAN_POINT('Ctrl Pts',(-6.20295651325157,0.179997595512823,
3.64190047202365));
#13133=CARTESIAN_POINT('Ctrl Pts',(-6.32432621115477,0.458374743512086,
3.65347812777622));
#13134=CARTESIAN_POINT('Ctrl Pts',(-6.53898438351643,0.672840241042802,
3.66504529364933));
#13135=CARTESIAN_POINT('Ctrl Pts',(-6.81680637706894,0.794134031701534,
3.67660197812095));
#13136=CARTESIAN_POINT('Ctrl Pts',(-7.11950248291682,0.805397533837699,
3.68814819174188));
#13137=CARTESIAN_POINT('Ctrl Pts',(-7.34163561569263,0.727628486768507,
3.69712044609008));
#13138=CARTESIAN_POINT('Ctrl Pts',(-7.53458281141515,0.599570945127131,
3.70608728556614));
#13139=CARTESIAN_POINT('Ctrl Pts',(-7.71503532521363,0.400461841999,3.71632891696956));
#13140=CARTESIAN_POINT('Ctrl Pts',(-7.82528743114405,0.0430926937144543,
3.73039630239659));
#13141=CARTESIAN_POINT('Ctrl Pts',(-7.74111169379658,-0.37323537543407,
3.74636272256909));
#13142=CARTESIAN_POINT('Ctrl Pts',(-7.44499573228645,-0.704767123835098,
3.76294659713056));
#13143=CARTESIAN_POINT('Ctrl Pts',(-7.00172600054551,-0.832350159693755,
3.78014508956006));
#13144=CARTESIAN_POINT('Ctrl Pts',(-6.55926311085665,-0.704755991680177,
3.79732045846001));
#13145=CARTESIAN_POINT('Ctrl Pts',(-6.2528315275211,-0.361772892660608,
3.81447281592693));
#13146=CARTESIAN_POINT('Ctrl Pts',(-6.17601189131465,0.0911409447444953,
3.83160228337755));
#13147=CARTESIAN_POINT('Ctrl Pts',(-6.35159897954253,0.514776986788965,
3.84870899394101));
#13148=CARTESIAN_POINT('Ctrl Pts',(-6.72535286944806,0.780122083208515,
3.86579309179979));
#13149=CARTESIAN_POINT('Ctrl Pts',(-7.13122870473182,0.802254155922275,
3.88095899359145));
#13150=CARTESIAN_POINT('Ctrl Pts',(-7.44985202071078,0.662844517922881,
3.89421470788503));
#13151=CARTESIAN_POINT('Ctrl Pts',(-7.66049480984587,0.452421922662202,
3.90556689264628));
#13152=CARTESIAN_POINT('Ctrl Pts',(-7.77936222711058,0.179641079514188,
3.91690927461427));
#13153=CARTESIAN_POINT('Ctrl Pts',(-7.79055864897702,-0.117447939280878,
3.92824190893221));
#13154=CARTESIAN_POINT('Ctrl Pts',(-7.69235883457516,-0.397692735498425,
3.93956485365948));
#13155=CARTESIAN_POINT('Ctrl Pts',(-7.4988193112063,-0.622862064421365,
3.95087816922642));
#13156=CARTESIAN_POINT('Ctrl Pts',(-7.23669309425985,-0.760857052520071,
3.96218191668704));
#13157=CARTESIAN_POINT('Ctrl Pts',(-6.84397122474983,-0.806385392143749,
3.97724090685452));
#13158=CARTESIAN_POINT('Ctrl Pts',(-6.3759149329141,-0.581575494059258,
3.99604104936904));
#13159=CARTESIAN_POINT('Ctrl Pts',(-6.14801487092373,-0.00140577011587543,
4.01856401164168));
#13160=CARTESIAN_POINT('Ctrl Pts',(-6.37569406553146,0.577216837917985,
4.04105035155356));
#13161=CARTESIAN_POINT('Ctrl Pts',(-6.93503804704956,0.846504117962824,
4.06350067666592));
#13162=CARTESIAN_POINT('Ctrl Pts',(-7.52735353249786,0.663517124905538,
4.08591563261074));
#13163=CARTESIAN_POINT('Ctrl Pts',(-7.83667549320556,0.127633503183688,
4.10829588960443));
#13164=CARTESIAN_POINT('Ctrl Pts',(-7.69892862810743,-0.475216209100622,
4.13064214875721));
#13165=CARTESIAN_POINT('Ctrl Pts',(-7.24587822138796,-0.783213519985818,
4.15047591997482));
#13166=CARTESIAN_POINT('Ctrl Pts',(-6.78448909503242,-0.770150049272615,
4.16780939837816));
#13167=CARTESIAN_POINT('Ctrl Pts',(-6.44291255401028,-0.573358437418835,
4.18265244830762));
#13168=CARTESIAN_POINT('Ctrl Pts',(-6.23727444607057,-0.236582538920206,
4.19748151807985));
#13169=CARTESIAN_POINT('Ctrl Pts',(-6.21750233201011,0.156779347523281,
4.21229685032696));
#13170=CARTESIAN_POINT('Ctrl Pts',(-6.38851989967645,0.511421035774412,
4.22709868951428));
#13171=CARTESIAN_POINT('Ctrl Pts',(-6.68127276436824,0.721655369840554,
4.24065490665371));
#13172=CARTESIAN_POINT('Ctrl Pts',(-6.99873870462004,0.781500222137114,
4.25296927229394));
#13173=CARTESIAN_POINT('Ctrl Pts',(-7.28423799128053,0.727580241858167,
4.26404501085876));
#13174=CARTESIAN_POINT('Ctrl Pts',(-7.52996735384668,0.573044604556925,
4.27511366794562));
#13175=CARTESIAN_POINT('Ctrl Pts',(-7.70249233600175,0.339504000304913,
4.28617535676904));
#13176=CARTESIAN_POINT('Ctrl Pts',(-7.77704029199075,0.0596812865399207,
4.29723019232866));
#13177=CARTESIAN_POINT('Ctrl Pts',(-7.73493077249201,-0.32516426809182,
4.31196099263524));
#13178=CARTESIAN_POINT('Ctrl Pts',(-7.48195320169677,-0.642258532616097,
4.32667855077855));
#13179=CARTESIAN_POINT('Ctrl Pts',(-7.11676447072565,-0.768672906025829,
4.34138335007881));
#13180=CARTESIAN_POINT('Ctrl Pts',(-6.82822052968084,-0.75826459078673,
4.35240569057047));
#13181=CARTESIAN_POINT('Ctrl Pts',(-6.56324655367934,-0.642480501470498,
4.36342189483669));
#13182=CARTESIAN_POINT('Ctrl Pts',(-6.3590246126422,-0.438361948172784,
4.37443208856579));
#13183=CARTESIAN_POINT('Ctrl Pts',(-6.24366823031993,-0.173725992278803,
4.38543639651659));
#13184=CARTESIAN_POINT('Ctrl Pts',(-6.23278862096309,0.114603786226641,
4.39643494391794));
#13185=CARTESIAN_POINT('Ctrl Pts',(-6.32818140570146,0.3866727001158,4.40742785948479));
#13186=CARTESIAN_POINT('Ctrl Pts',(-6.54732728408833,0.641795528726263,
4.42024651101618));
#13187=CARTESIAN_POINT('Ctrl Pts',(-6.90966296029133,0.792450205988824,
4.43488744119146));
#13188=CARTESIAN_POINT('Ctrl Pts',(-7.34497884959273,0.718229352606656,
4.45134684847234));
#13189=CARTESIAN_POINT('Ctrl Pts',(-7.67373744220819,0.42439860304808,4.46779506017063));
#13190=CARTESIAN_POINT('Ctrl Pts',(-7.7957623026863,0.000795392209376382,
4.48423253597012));
#13191=CARTESIAN_POINT('Ctrl Pts',(-7.6737681501059,-0.422451523433032,
4.50065973137187));
#13192=CARTESIAN_POINT('Ctrl Pts',(-7.34550270887416,-0.715780174479536,
4.51707711746896));
#13193=CARTESIAN_POINT('Ctrl Pts',(-6.91173568096419,-0.789442989854855,
4.53348515869499));
#13194=CARTESIAN_POINT('Ctrl Pts',(-6.50548543634235,-0.62113576023861,
4.54988433137086));
#13195=CARTESIAN_POINT('Ctrl Pts',(-6.25117725190974,-0.26266942709969,
4.56627511486019));
#13196=CARTESIAN_POINT('Ctrl Pts',(-6.22657268391725,0.175941615799059,
4.58265798957595));
#13197=CARTESIAN_POINT('Ctrl Pts',(-6.43900037753832,0.560237327905976,
4.59903344336352));
#13198=CARTESIAN_POINT('Ctrl Pts',(-6.82315231070266,0.772532064615231,
4.61540196293227));
#13199=CARTESIAN_POINT('Ctrl Pts',(-7.2612181287951,0.747894614274433,4.63176404577646));
#13200=CARTESIAN_POINT('Ctrl Pts',(-7.61885424416052,0.494109349486934,
4.64812018315545));
#13201=CARTESIAN_POINT('Ctrl Pts',(-7.78669901230814,0.0889725746862699,
4.66447087596232));
#13202=CARTESIAN_POINT('Ctrl Pts',(-7.72532501848925,-0.270994143806812,
4.67809233336064));
#13203=CARTESIAN_POINT('Ctrl Pts',(-7.56738721688822,-0.506594326857297,
4.68898728035258));
#13204=CARTESIAN_POINT('Ctrl Pts',(-7.35097564028756,-0.689891456361417,
4.69988083117445));
#13205=CARTESIAN_POINT('Ctrl Pts',(-7.0003169174225,-0.79110738140522,4.71349530909451));
#13206=CARTESIAN_POINT('Ctrl Pts',(-6.57937611771461,-0.669773743535281,
4.72982925479887));
#13207=CARTESIAN_POINT('Ctrl Pts',(-6.28761734218788,-0.343284450620702,
4.74616028288309));
#13208=CARTESIAN_POINT('Ctrl Pts',(-6.21426971041073,0.0883871334668474,
4.76248890194073));
#13209=CARTESIAN_POINT('Ctrl Pts',(-6.38182100128212,0.492840639406237,
4.77881561989744));
#13210=CARTESIAN_POINT('Ctrl Pts',(-6.73884045313308,0.746153973023737,
4.79514095601288));
#13211=CARTESIAN_POINT('Ctrl Pts',(-7.17589338359863,0.770679755263529,
4.81146540426486));
#13212=CARTESIAN_POINT('Ctrl Pts',(-7.55900114520461,0.55894423669953,4.82778951061359));
#13213=CARTESIAN_POINT('Ctrl Pts',(-7.77075750409873,0.175788412965931,
4.84411370102291));
#13214=CARTESIAN_POINT('Ctrl Pts',(-7.74620736592161,-0.261233995076225,
4.86043866853608));
#13215=CARTESIAN_POINT('Ctrl Pts',(-7.49294321470503,-0.618448872812403,
4.87676449790797));
#13216=CARTESIAN_POINT('Ctrl Pts',(-7.08837163954946,-0.785730122461179,
4.89309260172666));
#13217=CARTESIAN_POINT('Ctrl Pts',(-6.65674407499508,-0.712671607108413,
4.90942182102584));
#13218=CARTESIAN_POINT('Ctrl Pts',(-6.33017289353631,-0.420518596063947,
4.92575590410514));
#13219=CARTESIAN_POINT('Ctrl Pts',(-6.2493887150478,-0.140566474730618,
4.93664355063335));
#13220=CARTESIAN_POINT('Ctrl Pts',(-6.24936976727053,0.000312488344807942,
4.94209250793942));
#13221=CARTESIAN_POINT('',(-6.20000025990999,0.00193246945643844,1.00003735833913));
#13222=CARTESIAN_POINT('Origin',(-6.2,-1.64817900953001E-18,1.05));
#13223=CARTESIAN_POINT('',(-6.24936976727053,0.000312488344807943,4.94209250793942));
#13224=CARTESIAN_POINT('Ctrl Pts',(-6.20000025990999,0.00193246945643844,
1.00003735833913));
#13225=CARTESIAN_POINT('Ctrl Pts',(-6.20002044487095,0.15201065585541,1.00584212579936));
#13226=CARTESIAN_POINT('Ctrl Pts',(-6.28611355781982,0.450654413607575,
1.01745595262984));
#13227=CARTESIAN_POINT('Ctrl Pts',(-6.63487773043299,0.762776896374944,
1.0349026678303));
#13228=CARTESIAN_POINT('Ctrl Pts',(-7.09661480461016,0.841046944166038,
1.05237210147879));
#13229=CARTESIAN_POINT('Ctrl Pts',(-7.5301000809641,0.66191148032223,1.06986555847399));
#13230=CARTESIAN_POINT('Ctrl Pts',(-7.8019176387512,0.278705057923738,1.08738232429735));
#13231=CARTESIAN_POINT('Ctrl Pts',(-7.82838413701279,-0.19084760704926,
1.10492270302733));
#13232=CARTESIAN_POINT('Ctrl Pts',(-7.60064075566285,-0.603137091155931,
1.12248646715818));
#13233=CARTESIAN_POINT('Ctrl Pts',(-7.1879122444388,-0.831327694844811,
1.1400736154085));
#13234=CARTESIAN_POINT('Ctrl Pts',(-6.71648331627183,-0.804952825733149,
1.15768402928987));
#13235=CARTESIAN_POINT('Ctrl Pts',(-6.33069129380762,-0.53139586788873,
1.17531762920689));
#13236=CARTESIAN_POINT('Ctrl Pts',(-6.17986938434826,-0.166924530929506,
1.19003152205635));
#13237=CARTESIAN_POINT('Ctrl Pts',(-6.18891827393114,0.139694417819641,
1.20181411747366));
#13238=CARTESIAN_POINT('Ctrl Pts',(-6.28167759636603,0.432287479563812,
1.21360434390419));
#13239=CARTESIAN_POINT('Ctrl Pts',(-6.54498491257115,0.727352514001043,
1.22835639528026));
#13240=CARTESIAN_POINT('Ctrl Pts',(-7.00178799837524,0.858989074734809,
1.2460815491715));
#13241=CARTESIAN_POINT('Ctrl Pts',(-7.45905640505002,0.727341633611197,
1.2638292469814));
#13242=CARTESIAN_POINT('Ctrl Pts',(-7.77665281049733,0.372097321399229,
1.28159932797245));
#13243=CARTESIAN_POINT('Ctrl Pts',(-7.85663990835041,-0.0982374580424732,
1.29939162334549));
#13244=CARTESIAN_POINT('Ctrl Pts',(-7.67391806687674,-0.539592338752092,
1.31720595246947));
#13245=CARTESIAN_POINT('Ctrl Pts',(-7.28390423314539,-0.816419475206943,
1.33504212338853));
#13246=CARTESIAN_POINT('Ctrl Pts',(-6.80581165670056,-0.843349744908527,
1.35289993632842));
#13247=CARTESIAN_POINT('Ctrl Pts',(-6.38616737126169,-0.61151281975725,
1.37077917836497));
#13248=CARTESIAN_POINT('Ctrl Pts',(-6.15391471330266,-0.191448545046746,
1.38867962991899));
#13249=CARTESIAN_POINT('Ctrl Pts',(-6.18078031189829,0.288356063072798,
1.40660105660474));
#13250=CARTESIAN_POINT('Ctrl Pts',(-6.45912099114284,0.680780452257456,
1.42454321935777));
#13251=CARTESIAN_POINT('Ctrl Pts',(-6.90408886634936,0.865172061566579,
1.44250586618275));
#13252=CARTESIAN_POINT('Ctrl Pts',(-7.37948719351768,0.784486199243698,
1.46048873474343));
#13253=CARTESIAN_POINT('Ctrl Pts',(-7.73949168252554,0.462850086060547,
1.47849155669373));
#13254=CARTESIAN_POINT('Ctrl Pts',(-7.87332738631526,-0.0014557841833066,
1.49651404939771));
#13255=CARTESIAN_POINT('Ctrl Pts',(-7.73949699110486,-0.466462821459191,
1.51455592727214));
#13256=CARTESIAN_POINT('Ctrl Pts',(-7.43853082628792,-0.735208997602771,
1.52960672657187));
#13257=CARTESIAN_POINT('Ctrl Pts',(-7.13950426621928,-0.830029799823059,
1.5416567556677));
#13258=CARTESIAN_POINT('Ctrl Pts',(-6.82573429908325,-0.839341203501555,
1.55371299076107));
#13259=CARTESIAN_POINT('Ctrl Pts',(-6.46884268588545,-0.691631510671627,
1.56812451918729));
#13260=CARTESIAN_POINT('Ctrl Pts',(-6.19953260950331,-0.335836989319061,
1.58489796930832));
#13261=CARTESIAN_POINT('Ctrl Pts',(-6.13558329245919,0.087838843174565,
1.60101457637617));
#13262=CARTESIAN_POINT('Ctrl Pts',(-6.28224419701691,0.490989051876738,
1.61714503893002));
#13263=CARTESIAN_POINT('Ctrl Pts',(-6.60413478737033,0.775061465279082,
1.63328911262099));
#13264=CARTESIAN_POINT('Ctrl Pts',(-7.02294084448011,0.870730250827747,
1.64944654818199));
#13265=CARTESIAN_POINT('Ctrl Pts',(-7.43707348216018,0.754258049077075,
1.66561709103637));
#13266=CARTESIAN_POINT('Ctrl Pts',(-7.74477169774561,0.453838654047166,
1.68180048156974));
#13267=CARTESIAN_POINT('Ctrl Pts',(-7.88680288613318,-0.003482702933719,
1.69979600813884));
#13268=CARTESIAN_POINT('Ctrl Pts',(-7.73694295256561,-0.521688074393446,
1.71960864643413));
#13269=CARTESIAN_POINT('Ctrl Pts',(-7.2579246797109,-0.866176668338957,
1.74124367709995));
#13270=CARTESIAN_POINT('Ctrl Pts',(-6.71798257071652,-0.843361624137061,
1.76109465157299));
#13271=CARTESIAN_POINT('Ctrl Pts',(-6.32813840204838,-0.562067108424238,
1.779155502939));
#13272=CARTESIAN_POINT('Ctrl Pts',(-6.1403602470473,-0.172779460138823,
1.79542117132473));
#13273=CARTESIAN_POINT('Ctrl Pts',(-6.16191594592092,0.259681676239064,
1.81169744765855));
#13274=CARTESIAN_POINT('Ctrl Pts',(-6.38773509477738,0.629211178523826,
1.82798403284572));
#13275=CARTESIAN_POINT('Ctrl Pts',(-6.76298297690006,0.845905336791279,
1.84428062449289));
#13276=CARTESIAN_POINT('Ctrl Pts',(-7.1966047520639,0.856877177797125,1.86058691436274));
#13277=CARTESIAN_POINT('Ctrl Pts',(-7.51813159987616,0.691704323104765,
1.87418331464002));
#13278=CARTESIAN_POINT('Ctrl Pts',(-7.70496340534196,0.479537214773933,
1.88506497141452));
#13279=CARTESIAN_POINT('Ctrl Pts',(-7.834243376472,0.228058843588403,1.89594960161061));
#13280=CARTESIAN_POINT('Ctrl Pts',(-7.87040214071621,-0.132058080538115,
1.90956086256863));
#13281=CARTESIAN_POINT('Ctrl Pts',(-7.70176729712619,-0.532544739489079,
1.92590281458038));
#13282=CARTESIAN_POINT('Ctrl Pts',(-7.3617541753632,-0.803795766305812,
1.94225288140178));
#13283=CARTESIAN_POINT('Ctrl Pts',(-6.96910081682361,-0.872691342258758,
1.95724758038991));
#13284=CARTESIAN_POINT('Ctrl Pts',(-6.62358365553027,-0.779878922686934,
1.97088456464667));
#13285=CARTESIAN_POINT('Ctrl Pts',(-6.36438571820951,-0.588772954661729,
1.98316190508021));
#13286=CARTESIAN_POINT('Ctrl Pts',(-6.19306544459119,-0.315928048614165,
1.99544316011942));
#13287=CARTESIAN_POINT('Ctrl Pts',(-6.13303928680132,0.000731296674565001,
2.00772818860116));
#13288=CARTESIAN_POINT('Ctrl Pts',(-6.19306246181983,0.31737131710264,2.02001684693935));
#13289=CARTESIAN_POINT('Ctrl Pts',(-6.36452596264878,0.590662777058206,
2.03230899246722));
#13290=CARTESIAN_POINT('Ctrl Pts',(-6.62407285476001,0.781608449704824,
2.04460448181281));
#13291=CARTESIAN_POINT('Ctrl Pts',(-7.03960726862712,0.894452101215339,
2.06100273047082));
#13292=CARTESIAN_POINT('Ctrl Pts',(-7.58098213708746,0.728278840923384,
2.08150817561209));
#13293=CARTESIAN_POINT('Ctrl Pts',(-7.9216670182819,0.138324035331395,2.10612575173056));
#13294=CARTESIAN_POINT('Ctrl Pts',(-7.77006105183817,-0.525438678362505,
2.13075319116009));
#13295=CARTESIAN_POINT('Ctrl Pts',(-7.20723620509449,-0.909325593088126,
2.15538930422495));
#13296=CARTESIAN_POINT('Ctrl Pts',(-6.53333888373858,-0.807749099412924,
2.18003289797092));
#13297=CARTESIAN_POINT('Ctrl Pts',(-6.1083188432114,-0.274839326778277,
2.204682767912));
#13298=CARTESIAN_POINT('Ctrl Pts',(-6.15924265883207,0.405062095085805,
2.22933770998693));
#13299=CARTESIAN_POINT('Ctrl Pts',(-6.65910391363797,0.868885188693027,
2.25399651054932));
#13300=CARTESIAN_POINT('Ctrl Pts',(-7.34108037988483,0.868897827671466,
2.2786579570982));
#13301=CARTESIAN_POINT('Ctrl Pts',(-7.84103724749041,0.405011680967366,
2.30332083156262));
#13302=CARTESIAN_POINT('Ctrl Pts',(-7.89200269882987,-0.275103355231245,
2.32798391722886));
#13303=CARTESIAN_POINT('Ctrl Pts',(-7.46677961363602,-0.808302976870588,
2.35264599503351));
#13304=CARTESIAN_POINT('Ctrl Pts',(-6.79246102077101,-0.909925026569516,
2.37730584883283));
#13305=CARTESIAN_POINT('Ctrl Pts',(-6.22911235514946,-0.525814889228737,
2.40196226239673));
#13306=CARTESIAN_POINT('Ctrl Pts',(-6.07744456821118,0.138809074175696,
2.42661402385257));
#13307=CARTESIAN_POINT('Ctrl Pts',(-6.41824880300263,0.729027866722014,
2.45125992491537));
#13308=CARTESIAN_POINT('Ctrl Pts',(-7.06934122876124,0.929824149026898,
2.47589876067858));
#13309=CARTESIAN_POINT('Ctrl Pts',(-7.68299796183915,0.634246527935802,
2.50052933613646));
#13310=CARTESIAN_POINT('Ctrl Pts',(-7.93168967879738,0.000445263131447748,
2.52515045678013));
#13311=CARTESIAN_POINT('Ctrl Pts',(-7.68302213647328,-0.633094458923734,
2.54976094441856));
#13312=CARTESIAN_POINT('Ctrl Pts',(-7.07007700890629,-0.928102101680422,
2.57435962067245));
#13313=CARTESIAN_POINT('Ctrl Pts',(-6.42054771123064,-0.727833461900544,
2.59894532553828));
#13314=CARTESIAN_POINT('Ctrl Pts',(-6.08063030273252,-0.138905152375385,
2.62351690334527));
#13315=CARTESIAN_POINT('Ctrl Pts',(-6.20716604633801,0.411896009844242,
2.64398049630671));
#13316=CARTESIAN_POINT('Ctrl Pts',(-6.51199774209192,0.714676452673333,
2.66034317170459));
#13317=CARTESIAN_POINT('Ctrl Pts',(-6.80647130896726,0.843685013671235,
2.67261094147259));
#13318=CARTESIAN_POINT('Ctrl Pts',(-7.12812476587158,0.855502087711664,
2.68487433317324));
#13319=CARTESIAN_POINT('Ctrl Pts',(-7.43161948042588,0.749419002627999,
2.69713320958533));
#13320=CARTESIAN_POINT('Ctrl Pts',(-7.67521904640705,0.539636596661724,
2.7093874343511));
#13321=CARTESIAN_POINT('Ctrl Pts',(-7.82547325176268,0.255576344693996,
2.72163687040038));
#13322=CARTESIAN_POINT('Ctrl Pts',(-7.86123160253771,-0.0635635909156293,
2.73388138286896));
#13323=CARTESIAN_POINT('Ctrl Pts',(-7.76460027897753,-0.425533717492343,
2.74816074914963));
#13324=CARTESIAN_POINT('Ctrl Pts',(-7.47374360660769,-0.751894656156828,
2.76447137187111));
#13325=CARTESIAN_POINT('Ctrl Pts',(-7.00091436223893,-0.88782428734477,
2.78280870439184));
#13326=CARTESIAN_POINT('Ctrl Pts',(-6.52888862282209,-0.751805319722163,
2.80113347394993));
#13327=CARTESIAN_POINT('Ctrl Pts',(-6.2016684053735,-0.385612928895403,
2.81944525307317));
#13328=CARTESIAN_POINT('Ctrl Pts',(-6.11955382035284,0.0981170754742554,
2.83774361225262));
#13329=CARTESIAN_POINT('Ctrl Pts',(-6.30722625617569,0.551073055321834,
2.85602813457377));
#13330=CARTESIAN_POINT('Ctrl Pts',(-6.70680747045044,0.834525970819447,
2.87429840546262));
#13331=CARTESIAN_POINT('Ctrl Pts',(-7.19559869716282,0.861909407171868,
2.8925540164347));
#13332=CARTESIAN_POINT('Ctrl Pts',(-7.62360216624703,0.625277985438662,
2.91079457296321));
#13333=CARTESIAN_POINT('Ctrl Pts',(-7.86012925287909,0.197486531354187,
2.92901967711976));
#13334=CARTESIAN_POINT('Ctrl Pts',(-7.83237012712838,-0.289941720567784,
2.94722894753945));
#13335=CARTESIAN_POINT('Ctrl Pts',(-7.55008001741224,-0.687784692046307,
2.96542200407487));
#13336=CARTESIAN_POINT('Ctrl Pts',(-7.09977586824996,-0.874247976731781,
2.98359847915852));
#13337=CARTESIAN_POINT('Ctrl Pts',(-6.61974323779859,-0.792623075615972,
3.00175800933));
#13338=CARTESIAN_POINT('Ctrl Pts',(-6.257058130519,-0.468413543112272,3.0199002388146));
#13339=CARTESIAN_POINT('Ctrl Pts',(-6.12258713457564,-0.00138700255432796,
3.03802482606703));
#13340=CARTESIAN_POINT('Ctrl Pts',(-6.25706727378645,0.465139317147603,
3.05613142853581));
#13341=CARTESIAN_POINT('Ctrl Pts',(-6.61877666867083,0.788285032559405,
3.07421972093098));
#13342=CARTESIAN_POINT('Ctrl Pts',(-7.09647607914372,0.869376408975484,
3.09228937996591));
#13343=CARTESIAN_POINT('Ctrl Pts',(-7.54362920385282,0.68408153123717,3.11034009649877));
#13344=CARTESIAN_POINT('Ctrl Pts',(-7.82336210739947,0.28970919078182,3.12837156650594));
#13345=CARTESIAN_POINT('Ctrl Pts',(-7.85036951729978,-0.192518648808231,
3.1463834953635));
#13346=CARTESIAN_POINT('Ctrl Pts',(-7.61693284376151,-0.614735291409423,
3.16437560200786));
#13347=CARTESIAN_POINT('Ctrl Pts',(-7.19511476226595,-0.847778676228102,
3.18234760781168));
#13348=CARTESIAN_POINT('Ctrl Pts',(-6.7145098999882,-0.820710857786535,
3.20029925009486));
#13349=CARTESIAN_POINT('Ctrl Pts',(-6.32242256217712,-0.542413764760527,
3.21823027098919));
#13350=CARTESIAN_POINT('Ctrl Pts',(-6.13871066850024,-0.098686345015634,
3.23614042632575));
#13351=CARTESIAN_POINT('Ctrl Pts',(-6.21914065946509,0.374211025419683,
3.25402947870679));
#13352=CARTESIAN_POINT('Ctrl Pts',(-6.53845875539302,0.731406338297415,
3.27189720144838));
#13353=CARTESIAN_POINT('Ctrl Pts',(-6.99831755296742,0.863804065639348,
3.2897433804432));
#13354=CARTESIAN_POINT('Ctrl Pts',(-7.45757029965599,0.731409466469204,
3.30756780748229));
#13355=CARTESIAN_POINT('Ctrl Pts',(-7.77559982146972,0.37540881511312,3.32537028850097));
#13356=CARTESIAN_POINT('Ctrl Pts',(-7.85537931424834,-0.094642652826617,
3.34315063708933));
#13357=CARTESIAN_POINT('Ctrl Pts',(-7.67307624395954,-0.534539169893111,
3.36090867961867));
#13358=CARTESIAN_POINT('Ctrl Pts',(-7.28516805861167,-0.809670332991083,
3.37864425091963));
#13359=CARTESIAN_POINT('Ctrl Pts',(-6.81094328129299,-0.836216654728318,
3.39635719733567));
#13360=CARTESIAN_POINT('Ctrl Pts',(-6.39581795219668,-0.606687244699812,
3.41404737686194));
#13361=CARTESIAN_POINT('Ctrl Pts',(-6.16673282986248,-0.192016386472062,
3.43171465630725));
#13362=CARTESIAN_POINT('Ctrl Pts',(-6.19335105955753,0.280356102113162,
3.44935891493111));
#13363=CARTESIAN_POINT('Ctrl Pts',(-6.46683379484748,0.665660108445628,
3.46698004190314));
#13364=CARTESIAN_POINT('Ctrl Pts',(-6.90284795213186,0.846152102600437,
3.48457793824716));
#13365=CARTESIAN_POINT('Ctrl Pts',(-7.36737219772646,0.767129205800447,
3.50215251490095));
#13366=CARTESIAN_POINT('Ctrl Pts',(-7.71834143496065,0.453434200086869,
3.51970369457236));
#13367=CARTESIAN_POINT('Ctrl Pts',(-7.82645846631761,0.077080609195679,
3.53431012488451));
#13368=CARTESIAN_POINT('Ctrl Pts',(-7.78351602643939,-0.223766099777631,
3.54598350983127));
#13369=CARTESIAN_POINT('Ctrl Pts',(-7.65984666406284,-0.501195016191524,
3.55764904771478));
#13370=CARTESIAN_POINT('Ctrl Pts',(-7.36883520137935,-0.761421141511966,
3.57221624328425));
#13371=CARTESIAN_POINT('Ctrl Pts',(-6.90699782821215,-0.839986918687281,
3.58967328199228));
#13372=CARTESIAN_POINT('Ctrl Pts',(-6.5235772119384,-0.680444831465126,
3.60516965595896));
#13373=CARTESIAN_POINT('Ctrl Pts',(-6.29205860881578,-0.410854643842501,
3.6187136684483));
#13374=CARTESIAN_POINT('Ctrl Pts',(-6.19144251696091,-0.123792268925567,
3.63031232027941));
#13375=CARTESIAN_POINT('Ctrl Pts',(-6.20295651325157,0.179997595512823,
3.64190047202365));
#13376=CARTESIAN_POINT('Ctrl Pts',(-6.32432621115477,0.458374743512086,
3.65347812777622));
#13377=CARTESIAN_POINT('Ctrl Pts',(-6.53898438351643,0.672840241042802,
3.66504529364933));
#13378=CARTESIAN_POINT('Ctrl Pts',(-6.81680637706894,0.794134031701534,
3.67660197812095));
#13379=CARTESIAN_POINT('Ctrl Pts',(-7.11950248291682,0.805397533837699,
3.68814819174188));
#13380=CARTESIAN_POINT('Ctrl Pts',(-7.34163561569263,0.727628486768507,
3.69712044609008));
#13381=CARTESIAN_POINT('Ctrl Pts',(-7.53458281141515,0.599570945127131,
3.70608728556614));
#13382=CARTESIAN_POINT('Ctrl Pts',(-7.71503532521363,0.400461841999,3.71632891696956));
#13383=CARTESIAN_POINT('Ctrl Pts',(-7.82528743114405,0.0430926937144543,
3.73039630239659));
#13384=CARTESIAN_POINT('Ctrl Pts',(-7.74111169379658,-0.37323537543407,
3.74636272256909));
#13385=CARTESIAN_POINT('Ctrl Pts',(-7.44499573228645,-0.704767123835098,
3.76294659713056));
#13386=CARTESIAN_POINT('Ctrl Pts',(-7.00172600054551,-0.832350159693755,
3.78014508956006));
#13387=CARTESIAN_POINT('Ctrl Pts',(-6.55926311085665,-0.704755991680177,
3.79732045846001));
#13388=CARTESIAN_POINT('Ctrl Pts',(-6.2528315275211,-0.361772892660608,
3.81447281592693));
#13389=CARTESIAN_POINT('Ctrl Pts',(-6.17601189131465,0.0911409447444953,
3.83160228337755));
#13390=CARTESIAN_POINT('Ctrl Pts',(-6.35159897954253,0.514776986788965,
3.84870899394101));
#13391=CARTESIAN_POINT('Ctrl Pts',(-6.72535286944806,0.780122083208515,
3.86579309179979));
#13392=CARTESIAN_POINT('Ctrl Pts',(-7.13122870473182,0.802254155922275,
3.88095899359145));
#13393=CARTESIAN_POINT('Ctrl Pts',(-7.44985202071078,0.662844517922881,
3.89421470788503));
#13394=CARTESIAN_POINT('Ctrl Pts',(-7.66049480984587,0.452421922662202,
3.90556689264628));
#13395=CARTESIAN_POINT('Ctrl Pts',(-7.77936222711058,0.179641079514188,
3.91690927461427));
#13396=CARTESIAN_POINT('Ctrl Pts',(-7.79055864897702,-0.117447939280878,
3.92824190893221));
#13397=CARTESIAN_POINT('Ctrl Pts',(-7.69235883457516,-0.397692735498425,
3.93956485365948));
#13398=CARTESIAN_POINT('Ctrl Pts',(-7.4988193112063,-0.622862064421365,
3.95087816922642));
#13399=CARTESIAN_POINT('Ctrl Pts',(-7.23669309425985,-0.760857052520071,
3.96218191668704));
#13400=CARTESIAN_POINT('Ctrl Pts',(-6.84397122474983,-0.806385392143749,
3.97724090685452));
#13401=CARTESIAN_POINT('Ctrl Pts',(-6.3759149329141,-0.581575494059258,
3.99604104936904));
#13402=CARTESIAN_POINT('Ctrl Pts',(-6.14801487092373,-0.00140577011587543,
4.01856401164168));
#13403=CARTESIAN_POINT('Ctrl Pts',(-6.37569406553146,0.577216837917985,
4.04105035155356));
#13404=CARTESIAN_POINT('Ctrl Pts',(-6.93503804704956,0.846504117962824,
4.06350067666592));
#13405=CARTESIAN_POINT('Ctrl Pts',(-7.52735353249786,0.663517124905538,
4.08591563261074));
#13406=CARTESIAN_POINT('Ctrl Pts',(-7.83667549320556,0.127633503183688,
4.10829588960443));
#13407=CARTESIAN_POINT('Ctrl Pts',(-7.69892862810743,-0.475216209100622,
4.13064214875721));
#13408=CARTESIAN_POINT('Ctrl Pts',(-7.24587822138796,-0.783213519985818,
4.15047591997482));
#13409=CARTESIAN_POINT('Ctrl Pts',(-6.78448909503242,-0.770150049272615,
4.16780939837816));
#13410=CARTESIAN_POINT('Ctrl Pts',(-6.44291255401028,-0.573358437418835,
4.18265244830762));
#13411=CARTESIAN_POINT('Ctrl Pts',(-6.23727444607057,-0.236582538920206,
4.19748151807985));
#13412=CARTESIAN_POINT('Ctrl Pts',(-6.21750233201011,0.156779347523281,
4.21229685032696));
#13413=CARTESIAN_POINT('Ctrl Pts',(-6.38851989967645,0.511421035774412,
4.22709868951428));
#13414=CARTESIAN_POINT('Ctrl Pts',(-6.68127276436824,0.721655369840554,
4.24065490665371));
#13415=CARTESIAN_POINT('Ctrl Pts',(-6.99873870462004,0.781500222137114,
4.25296927229394));
#13416=CARTESIAN_POINT('Ctrl Pts',(-7.28423799128053,0.727580241858167,
4.26404501085876));
#13417=CARTESIAN_POINT('Ctrl Pts',(-7.52996735384668,0.573044604556925,
4.27511366794562));
#13418=CARTESIAN_POINT('Ctrl Pts',(-7.70249233600175,0.339504000304913,
4.28617535676904));
#13419=CARTESIAN_POINT('Ctrl Pts',(-7.77704029199075,0.0596812865399207,
4.29723019232866));
#13420=CARTESIAN_POINT('Ctrl Pts',(-7.73493077249201,-0.32516426809182,
4.31196099263524));
#13421=CARTESIAN_POINT('Ctrl Pts',(-7.48195320169677,-0.642258532616097,
4.32667855077855));
#13422=CARTESIAN_POINT('Ctrl Pts',(-7.11676447072565,-0.768672906025829,
4.34138335007881));
#13423=CARTESIAN_POINT('Ctrl Pts',(-6.82822052968084,-0.75826459078673,
4.35240569057047));
#13424=CARTESIAN_POINT('Ctrl Pts',(-6.56324655367934,-0.642480501470498,
4.36342189483669));
#13425=CARTESIAN_POINT('Ctrl Pts',(-6.3590246126422,-0.438361948172784,
4.37443208856579));
#13426=CARTESIAN_POINT('Ctrl Pts',(-6.24366823031993,-0.173725992278803,
4.38543639651659));
#13427=CARTESIAN_POINT('Ctrl Pts',(-6.23278862096309,0.114603786226641,
4.39643494391794));
#13428=CARTESIAN_POINT('Ctrl Pts',(-6.32818140570146,0.3866727001158,4.40742785948479));
#13429=CARTESIAN_POINT('Ctrl Pts',(-6.54732728408833,0.641795528726263,
4.42024651101618));
#13430=CARTESIAN_POINT('Ctrl Pts',(-6.90966296029133,0.792450205988824,
4.43488744119146));
#13431=CARTESIAN_POINT('Ctrl Pts',(-7.34497884959273,0.718229352606656,
4.45134684847234));
#13432=CARTESIAN_POINT('Ctrl Pts',(-7.67373744220819,0.42439860304808,4.46779506017063));
#13433=CARTESIAN_POINT('Ctrl Pts',(-7.7957623026863,0.000795392209376382,
4.48423253597012));
#13434=CARTESIAN_POINT('Ctrl Pts',(-7.6737681501059,-0.422451523433032,
4.50065973137187));
#13435=CARTESIAN_POINT('Ctrl Pts',(-7.34550270887416,-0.715780174479536,
4.51707711746896));
#13436=CARTESIAN_POINT('Ctrl Pts',(-6.91173568096419,-0.789442989854855,
4.53348515869499));
#13437=CARTESIAN_POINT('Ctrl Pts',(-6.50548543634235,-0.62113576023861,
4.54988433137086));
#13438=CARTESIAN_POINT('Ctrl Pts',(-6.25117725190974,-0.26266942709969,
4.56627511486019));
#13439=CARTESIAN_POINT('Ctrl Pts',(-6.22657268391725,0.175941615799059,
4.58265798957595));
#13440=CARTESIAN_POINT('Ctrl Pts',(-6.43900037753832,0.560237327905976,
4.59903344336352));
#13441=CARTESIAN_POINT('Ctrl Pts',(-6.82315231070266,0.772532064615231,
4.61540196293227));
#13442=CARTESIAN_POINT('Ctrl Pts',(-7.2612181287951,0.747894614274433,4.63176404577646));
#13443=CARTESIAN_POINT('Ctrl Pts',(-7.61885424416052,0.494109349486934,
4.64812018315545));
#13444=CARTESIAN_POINT('Ctrl Pts',(-7.78669901230814,0.0889725746862699,
4.66447087596232));
#13445=CARTESIAN_POINT('Ctrl Pts',(-7.72532501848925,-0.270994143806812,
4.67809233336064));
#13446=CARTESIAN_POINT('Ctrl Pts',(-7.56738721688822,-0.506594326857297,
4.68898728035258));
#13447=CARTESIAN_POINT('Ctrl Pts',(-7.35097564028756,-0.689891456361417,
4.69988083117445));
#13448=CARTESIAN_POINT('Ctrl Pts',(-7.0003169174225,-0.79110738140522,4.71349530909451));
#13449=CARTESIAN_POINT('Ctrl Pts',(-6.57937611771461,-0.669773743535281,
4.72982925479887));
#13450=CARTESIAN_POINT('Ctrl Pts',(-6.28761734218788,-0.343284450620702,
4.74616028288309));
#13451=CARTESIAN_POINT('Ctrl Pts',(-6.21426971041073,0.0883871334668474,
4.76248890194073));
#13452=CARTESIAN_POINT('Ctrl Pts',(-6.38182100128212,0.492840639406237,
4.77881561989744));
#13453=CARTESIAN_POINT('Ctrl Pts',(-6.73884045313308,0.746153973023737,
4.79514095601288));
#13454=CARTESIAN_POINT('Ctrl Pts',(-7.17589338359863,0.770679755263529,
4.81146540426486));
#13455=CARTESIAN_POINT('Ctrl Pts',(-7.55900114520461,0.55894423669953,4.82778951061359));
#13456=CARTESIAN_POINT('Ctrl Pts',(-7.77075750409873,0.175788412965931,
4.84411370102291));
#13457=CARTESIAN_POINT('Ctrl Pts',(-7.74620736592161,-0.261233995076225,
4.86043866853608));
#13458=CARTESIAN_POINT('Ctrl Pts',(-7.49294321470503,-0.618448872812403,
4.87676449790797));
#13459=CARTESIAN_POINT('Ctrl Pts',(-7.08837163954946,-0.785730122461179,
4.89309260172666));
#13460=CARTESIAN_POINT('Ctrl Pts',(-6.65674407499508,-0.712671607108413,
4.90942182102584));
#13461=CARTESIAN_POINT('Ctrl Pts',(-6.33017289353631,-0.420518596063947,
4.92575590410514));
#13462=CARTESIAN_POINT('Ctrl Pts',(-6.2493887150478,-0.140566474730618,
4.93664355063335));
#13463=CARTESIAN_POINT('Ctrl Pts',(-6.24936976727053,0.000312488344807942,
4.94209250793942));
#13464=CARTESIAN_POINT('Origin',(-6.2,-3.91353616180368E-15,4.95));
#13465=CARTESIAN_POINT('Origin',(-6.2,-3.91353616180368E-15,4.95));
#13466=CARTESIAN_POINT('Origin',(-6.2,-1.64817900953001E-18,1.05));
#14977=UNCERTAINTY_MEASURE_WITH_UNIT(LENGTH_MEASURE(0.001),#15041,
'DISTANCE_ACCURACY_VALUE',
'Maximum model space distance between geometric entities at asserted c
onnectivities');
#15000=UNCERTAINTY_MEASURE_WITH_UNIT(LENGTH_MEASURE(0.001),#15041,
'DISTANCE_ACCURACY_VALUE',
'Maximum model space distance between geometric entities at asserted c
onnectivities');
#15017=(
GEOMETRIC_REPRESENTATION_CONTEXT(3)
GLOBAL_UNCERTAINTY_ASSIGNED_CONTEXT((#14977))
GLOBAL_UNIT_ASSIGNED_CONTEXT((#15041,#15043,#15044))
REPRESENTATION_CONTEXT('','3D')
);
#15040=(
GEOMETRIC_REPRESENTATION_CONTEXT(3)
GLOBAL_UNCERTAINTY_ASSIGNED_CONTEXT((#15000))
GLOBAL_UNIT_ASSIGNED_CONTEXT((#15041,#15043,#15044))
REPRESENTATION_CONTEXT('','3D')
);
#15041=(
LENGTH_UNIT()
NAMED_UNIT(*)
SI_UNIT(.CENTI.,.METRE.)
);
#15043=(
NAMED_UNIT(*)
PLANE_ANGLE_UNIT()
SI_UNIT($,.RADIAN.)
);
#15044=(
NAMED_UNIT(*)
SI_UNIT($,.STERADIAN.)
SOLID_ANGLE_UNIT()
);
#15061=SHAPE_DEFINITION_REPRESENTATION(#15100,#15198);
#15100=PRODUCT_DEFINITION_SHAPE('',$,#15238);
#15198=SHAPE_REPRESENTATION('',(#7703),#15017);
#15221=PRODUCT_DEFINITION_CONTEXT('part definition',#15340,'design');
#15238=PRODUCT_DEFINITION('Installed compression spring',
'Installed compression spring',#15277,#15221);
#15277=PRODUCT_DEFINITION_FORMATION('',$,#15358);
#15340=APPLICATION_CONTEXT(
'Core Data for Automotive Mechanical Design Process');
#15341=PRODUCT_CONTEXT('part definition',#15340,'mechanical');
#15358=PRODUCT('Installed compression spring',
'Installed compression spring','Installed compression spring',(#15341));
#15451=COLOUR_RGB('Grey',0.48,0.52,0.57);
#15452=FILL_AREA_STYLE_COLOUR('',#15451);
#15453=FILL_AREA_STYLE('',(#15452));
#15454=SURFACE_STYLE_FILL_AREA(#15453);
#15455=SURFACE_SIDE_STYLE('',(#15454));
#15456=SURFACE_STYLE_USAGE(.BOTH.,#15455);
#15457=PRESENTATION_STYLE_ASSIGNMENT((#15456));
ENDSEC;
END-ISO-10303-21;
